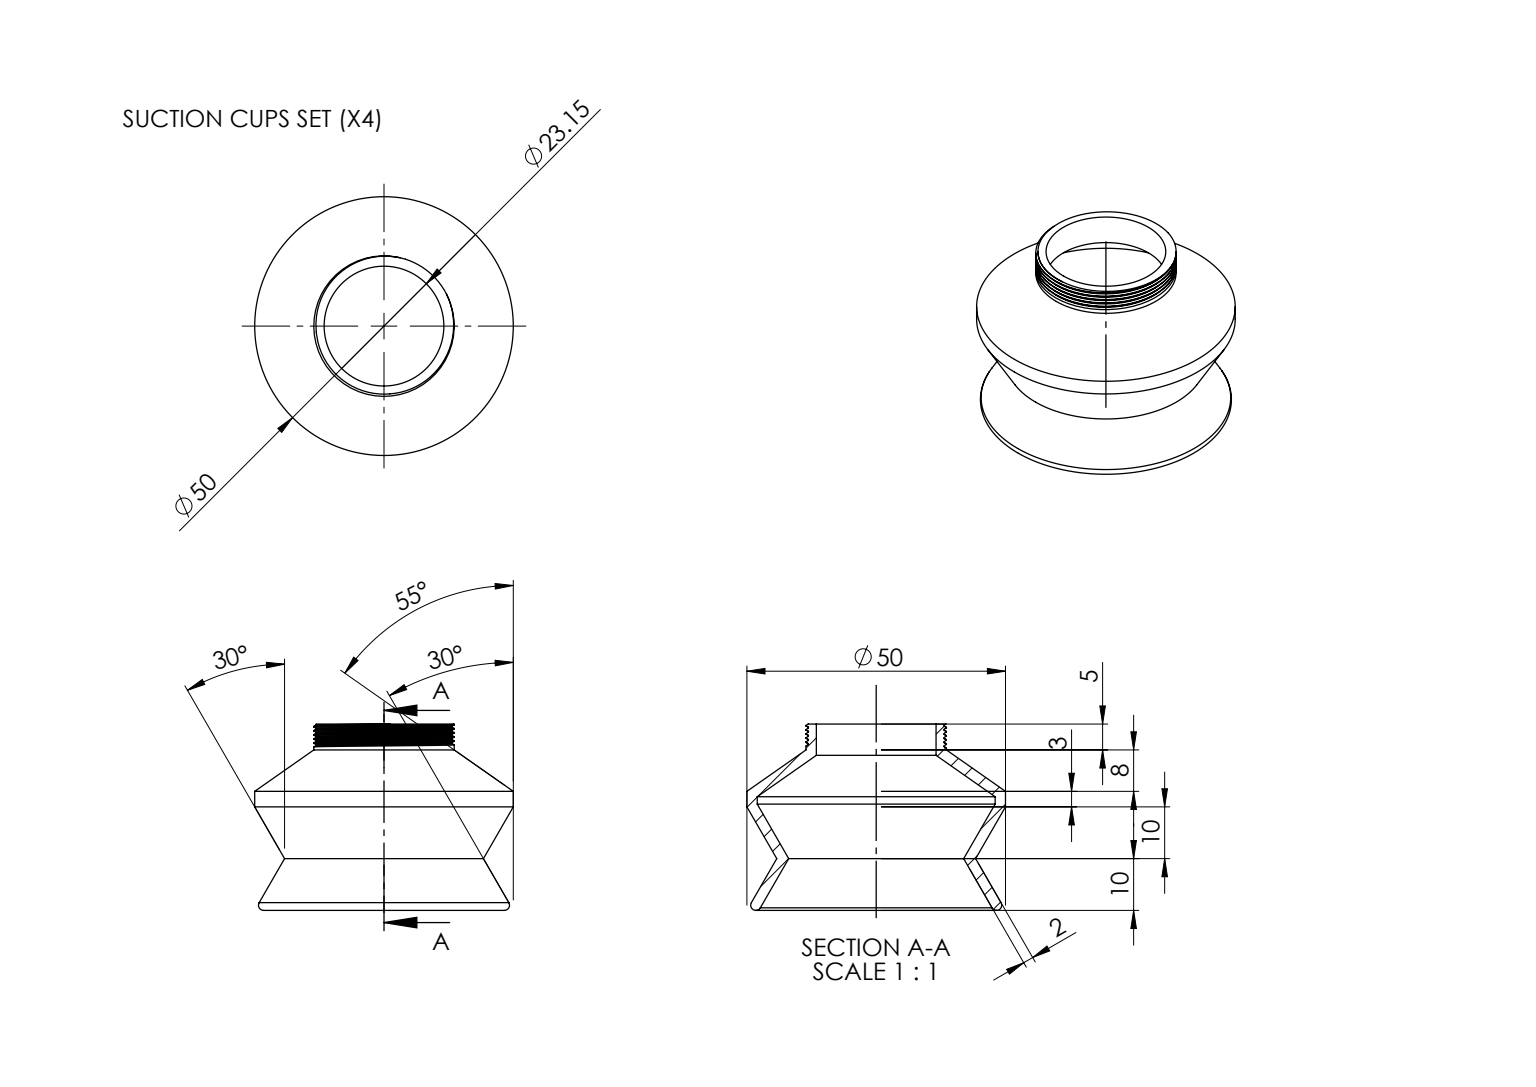
ISO-10303-21;
HEADER;
FILE_DESCRIPTION (('STEP AP214'),
    '1' );
FILE_NAME ('Suction Cups Set (x4).step',
    '2026-10-01T14:18:43',
    ( '' ),
    ( '' ),
    'SwSTEP 2.0',
    'SolidWorks 2026',
    '' );
FILE_SCHEMA (( 'AUTOMOTIVE_DESIGN' ));
ENDSEC;

DATA;
#7=ORIENTED_EDGE ( 'NONE', *, *, #7284, .F. ) ;
#8=CARTESIAN_POINT ( 'NONE',  ( 13.57481594606304753, 32.71523437500000142, -5.622872871577873966 ) ) ;
#12=CARTESIAN_POINT ( 'NONE',  ( 13.14518615778179544, 34.00507812608393721, -1.609821015232357215E-15 ) ) ;
#13=CARTESIAN_POINT ( 'NONE',  ( -5.444914386472299306, 39.31328125108394289, 13.14518615778179722 ) ) ;
#36=( BOUNDED_CURVE ( )  B_SPLINE_CURVE ( 2, ( #22936, #3397, #12350, #21068, #12069, #998, #12204, #16222, #18653 ),
 .UNSPECIFIED., .F., .F. ) 
 B_SPLINE_CURVE_WITH_KNOTS ( ( 3, 2, 2, 2, 3 ),
 ( 0.5208333333333332593, 0.5312499999999997780, 0.5416666666666664076, 0.5520833333333330373, 0.5624999999999996669 ),
 .UNSPECIFIED. ) 
 CURVE ( )  GEOMETRIC_REPRESENTATION_ITEM ( )  RATIONAL_B_SPLINE_CURVE ( ( 1.000000000000000888, 0.9238795325112859613, 1.000000000000000000, 0.9238795325112867385, 1.000000000000000000, 0.9238795325112867385, 1.000000000000000000, 0.9238795325112891810, 0.9999999999999975575 ) ) 
 REPRESENTATION_ITEM ( '' )  );
#41=CYLINDRICAL_SURFACE ( 'NONE', #26554, 13.57481594606304576 ) ;
#45=ORIENTED_EDGE ( 'NONE', *, *, #19075, .T. ) ;
#47=AXIS2_PLACEMENT_3D ( 'NONE', #20882, #18604, #27308 ) ;
#48=CARTESIAN_POINT ( 'NONE',  ( -13.14518615778179900, 40.50390625108394005, -5.444914386472297529 ) ) ;
#88=EDGE_CURVE ( 'NONE', #26327, #25494, #13051, .T. ) ;
#90=SURFACE_STYLE_USAGE ( .BOTH. , #4222 ) ;
#97=CARTESIAN_POINT ( 'NONE',  ( 13.14518615778179544, 38.56914062608393579, -1.609821015232357215E-15 ) ) ;
#113=DIRECTION ( 'NONE',  ( 0.000000000000000000, 0.000000000000000000, 1.000000000000000000 ) ) ;
#124=CARTESIAN_POINT ( 'NONE',  ( 13.57481594606304576, 37.42812499999999432, -1.662435489736055892E-15 ) ) ;
#126=CARTESIAN_POINT ( 'NONE',  ( 5.444914386472297529, 36.53515625108393294, -13.14518615778179900 ) ) ;
#148=ORIENTED_EDGE ( 'NONE', *, *, #16828, .T. ) ;
#149=CARTESIAN_POINT ( 'NONE',  ( -8.312177448680279460E-16, 32.96328125216787441, -13.57481594606304576 ) ) ;
#154=CARTESIAN_POINT ( 'NONE',  ( 13.14518615778179544, 38.76757812608393294, -1.609821015232357215E-15 ) ) ;
#233=CARTESIAN_POINT ( 'NONE',  ( 5.444914386472297529, 38.71796875108393721, -13.14518615778179900 ) ) ;
#244=ORIENTED_EDGE ( 'NONE', *, *, #571, .T. ) ;
#252=VECTOR ( 'NONE', #26544, 1000.000000000000114 ) ;
#253=CARTESIAN_POINT ( 'NONE',  ( 6.106658654948486920, 35.99999999999996447, 11.74215035806527396 ) ) ;
#266=CARTESIAN_POINT ( 'NONE',  ( -13.57481594606304576, 38.61874999999999147, 0.000000000000000000 ) ) ;
#268=CARTESIAN_POINT ( 'NONE',  ( 13.14518615778179900, 38.02343750108395426, -5.444914386472297529 ) ) ;
#281=ORIENTED_EDGE ( 'NONE', *, *, #3794, .F. ) ;
#285=TOROIDAL_SURFACE ( 'NONE', #12557, 23.26794919243112858, 1.000000000000000000 ) ;
#297=CARTESIAN_POINT ( 'NONE',  ( -9.295050272127046043, 39.06523437608392868, -9.295050272127046043 ) ) ;
#331=CARTESIAN_POINT ( 'NONE',  ( 13.14518615778179900, 38.51953125108393294, 5.444914386472293977 ) ) ;
#365=CARTESIAN_POINT ( 'NONE',  ( 2.493653234604083739E-15, 35.64218749999999147, 13.57481594606304576 ) ) ;
#380=CARTESIAN_POINT ( 'NONE',  ( -9.295050272127046043, 40.45429687608393721, -9.295050272127046043 ) ) ;
#391=ORIENTED_EDGE ( 'NONE', *, *, #1518, .F. ) ;
#399=ORIENTED_EDGE ( 'NONE', *, *, #6701, .T. ) ;
#400=CARTESIAN_POINT ( 'NONE',  ( 3.304118597822780057, 36.00000000000001421, 12.77244747738236441 ) ) ;
#409=CARTESIAN_POINT ( 'NONE',  ( -5.622872871578057818, 35.59257812499998863, 13.57481594606286457 ) ) ;
#411=CARTESIAN_POINT ( 'NONE',  ( -5.622872871577873077, 37.97382812499999716, 13.57481594606304753 ) ) ;
#413=CARTESIAN_POINT ( 'NONE',  ( -8.049105076161786076E-16, 36.58476562608393579, -13.14518615778179544 ) ) ;
#437=CARTESIAN_POINT ( 'NONE',  ( 5.444914386472297529, 35.74140625108393721, -13.14518615778179900 ) ) ;
#451=EDGE_CURVE ( 'NONE', #10079, #19989, #7039, .T. ) ;
#472=ORIENTED_EDGE ( 'NONE', *, *, #2653, .T. ) ;
#474=CARTESIAN_POINT ( 'NONE',  ( -13.14518615778179189, 39.01562500108393294, 5.444914386472304635 ) ) ;
#522=CARTESIAN_POINT ( 'NONE',  ( 13.14518615778179544, 35.39414062608393152, -1.609821015232357215E-15 ) ) ;
#554=CARTESIAN_POINT ( 'NONE',  ( 5.622872871577878406, 37.27929687499999289, 13.57481594606304576 ) ) ;
#555=CARTESIAN_POINT ( 'NONE',  ( -2.086998648631069653, 36.00000000000000000, -13.31420566034952202 ) ) ;
#556=CARTESIAN_POINT ( 'NONE',  ( -8.049105076161786076E-16, 33.40976562608393863, -13.14518615778179544 ) ) ;
#559=CARTESIAN_POINT ( 'NONE',  ( 9.598844408820459861, 35.04687500216787299, 9.598844408820456309 ) ) ;
#571=EDGE_CURVE ( 'NONE', #4666, #18529, #26293, .T. ) ;
#580=DIRECTION ( 'NONE',  ( 0.000000000000000000, 0.000000000000000000, -1.000000000000000000 ) ) ;
#584=CARTESIAN_POINT ( 'NONE',  ( -5.444914386472299306, 35.34453125108393579, 13.14518615778179722 ) ) ;
#615=CARTESIAN_POINT ( 'NONE',  ( 13.14518615778179900, 36.23750000108393010, -5.444914386472297529 ) ) ;
#645=ORIENTED_EDGE ( 'NONE', *, *, #3764, .T. ) ;
#658=CARTESIAN_POINT ( 'NONE',  ( -9.598844408820454532, 34.05468750216788010, 9.598844408820459861 ) ) ;
#660=ORIENTED_EDGE ( 'NONE', *, *, #2653, .F. ) ;
#664=CARTESIAN_POINT ( 'NONE',  ( -5.622872871577920151, 35.39414062716787868, -13.57481594606300135 ) ) ;
#667=CARTESIAN_POINT ( 'NONE',  ( -5.444914386472297529, 37.22968750108393721, -13.14518615778179900 ) ) ;
#690=CARTESIAN_POINT ( 'NONE',  ( -8.312177448680279460E-16, 37.72578125216787726, -13.57481594606304576 ) ) ;
#696=CARTESIAN_POINT ( 'NONE',  ( -9.598844408820458085, 35.34453124999998863, -9.598844408820458085 ) ) ;
#698=CARTESIAN_POINT ( 'NONE',  ( 5.622872871577878406, 34.10429687499999574, 13.57481594606304576 ) ) ;
#700=CARTESIAN_POINT ( 'NONE',  ( -13.14518615778179900, 33.55859375108393294, -5.444914386472297529 ) ) ;
#702=CARTESIAN_POINT ( 'NONE',  ( -9.295050272127044266, 35.09648437608392868, 9.295050272127047819 ) ) ;
#703=CARTESIAN_POINT ( 'NONE',  ( -5.622872871577873077, 34.89804687716787868, 13.57481594606304753 ) ) ;
#721=VECTOR ( 'NONE', #26504, 1000.000000000000000 ) ;
#727=CARTESIAN_POINT ( 'NONE',  ( 13.14518615778179900, 36.43593750108392726, -5.444914386472297529 ) ) ;
#733=EDGE_CURVE ( 'NONE', #12114, #10399, #2983, .T. ) ;
#743=AXIS2_PLACEMENT_3D ( 'NONE', #5650, #23447, #6063 ) ;
#750=DIRECTION ( 'NONE',  ( -1.000000000000000000, 0.000000000000000000, 0.000000000000000000 ) ) ;
#758=CARTESIAN_POINT ( 'NONE',  ( -13.14518615778179189, 35.04687500108393294, 5.444914386472304635 ) ) ;
#794=( BOUNDED_CURVE ( )  B_SPLINE_CURVE ( 2, ( #5981, #8244, #25772, #1851, #19221, #27923, #21502, #17214, #25918 ),
 .UNSPECIFIED., .F., .T. ) 
 B_SPLINE_CURVE_WITH_KNOTS ( ( 3, 2, 2, 2, 3 ),
 ( 0.5249747582430949189, 0.5312500000000001110, 0.5416666666666668517, 0.5520833333333337034, 0.5625000000000004441 ),
 .UNSPECIFIED. ) 
 CURVE ( )  GEOMETRIC_REPRESENTATION_ITEM ( )  RATIONAL_B_SPLINE_CURVE ( ( 0.9635368518655842429, 0.9541432637305302666, 1.000000000000000000, 0.9238795325112867385, 1.000000000000000000, 0.9238795325112867385, 1.000000000000000000, 0.9238795325112835188, 1.000000000000003331 ) ) 
 REPRESENTATION_ITEM ( '' )  );
#813=CARTESIAN_POINT ( 'NONE',  ( 2.414731522848535132E-15, 35.98945312608393010, 13.14518615778179544 ) ) ;
#837=CARTESIAN_POINT ( 'NONE',  ( -13.57481594606304576, 38.76757812716787299, 5.622872871577880183 ) ) ;
#845=CARTESIAN_POINT ( 'NONE',  ( -9.598844408820458085, 33.75703124999999005, -9.598844408820458085 ) ) ;
#847=CARTESIAN_POINT ( 'NONE',  ( 2.414731522848535132E-15, 35.39414062608393863, 13.14518615778179544 ) ) ;
#849=CARTESIAN_POINT ( 'NONE',  ( -13.14518615778179189, 34.25312500108393721, 5.444914386472304635 ) ) ;
#851=CARTESIAN_POINT ( 'NONE',  ( 13.57481594606304576, 35.14609375216787157, -1.662435489736055892E-15 ) ) ;
#876=CARTESIAN_POINT ( 'NONE',  ( -5.444914386472299306, 36.93203125108394147, 13.14518615778179722 ) ) ;
#906=CARTESIAN_POINT ( 'NONE',  ( 5.444914386472297529, 35.54296875108393294, -13.14518615778179900 ) ) ;
#908=CARTESIAN_POINT ( 'NONE',  ( 0.000000000000000000, 11.00000000000000355, 0.000000000000000000 ) ) ;
#909=CIRCLE ( 'NONE', #6776, 11.57481594606304576 ) ;
#963=ORIENTED_EDGE ( 'NONE', *, *, #21718, .F. ) ;
#977=CARTESIAN_POINT ( 'NONE',  ( 5.444914386472302859, 32.26875000108393721, 13.14518615778179189 ) ) ;
#980=CARTESIAN_POINT ( 'NONE',  ( -13.57481594606304576, 38.71796875216787726, 0.000000000000000000 ) ) ;
#984=EDGE_CURVE ( 'NONE', #27010, #13376, #11532, .T. ) ;
#988=CARTESIAN_POINT ( 'NONE',  ( 9.598844408820456309, 32.76484374999999716, -9.598844408820458085 ) ) ;
#990=CARTESIAN_POINT ( 'NONE',  ( 13.14518615778179544, 35.59257812608393579, -1.609821015232357215E-15 ) ) ;
#992=CARTESIAN_POINT ( 'NONE',  ( 9.295050272127046043, 35.49335937608393010, -9.295050272127046043 ) ) ;
#993=CARTESIAN_POINT ( 'NONE',  ( 13.57481594606304753, 36.78320312716786589, -5.622872871577873077 ) ) ;
#998=CARTESIAN_POINT ( 'NONE',  ( 13.57481594606304931, 35.09648437716787583, 5.622872871577868636 ) ) ;
#1019=CARTESIAN_POINT ( 'NONE',  ( 13.14518615778179900, 37.92421875108392726, 5.444914386472293977 ) ) ;
#1029=CARTESIAN_POINT ( 'NONE',  ( -5.622872871578010745, 32.91367187499999858, -13.57481594606290898 ) ) ;
#1048=CARTESIAN_POINT ( 'NONE',  ( -5.444914386472299306, 35.93984375108392726, 13.14518615778179722 ) ) ;
#1107=EDGE_LOOP ( 'NONE', ( #12800, #23533, #16863, #391 ) ) ;
#1116=CARTESIAN_POINT ( 'NONE',  ( 13.14518615778179722, 32.36796875108393579, 5.444914386472293977 ) ) ;
#1120=CARTESIAN_POINT ( 'NONE',  ( -9.598844408820454532, 39.61093750216787868, 9.598844408820459861 ) ) ;
#1121=CARTESIAN_POINT ( 'NONE',  ( 0.000000000000000000, 36.00000000000000000, 0.000000000000000000 ) ) ;
#1123=CARTESIAN_POINT ( 'NONE',  ( 2.493653234604083739E-15, 33.36015625216786873, 13.57481594606304576 ) ) ;
#1128=CARTESIAN_POINT ( 'NONE',  ( 13.57481594606304931, 34.99726562500000426, 5.622872871577869525 ) ) ;
#1130=CARTESIAN_POINT ( 'NONE',  ( -13.14518615778179544, 33.60820312608393579, 0.000000000000000000 ) ) ;
#1133=CARTESIAN_POINT ( 'NONE',  ( -8.049105076161786076E-16, 35.59257812608393579, -13.14518615778179544 ) ) ;
#1134=CARTESIAN_POINT ( 'NONE',  ( 9.598844408820456309, 35.24531250216787726, -9.598844408820458085 ) ) ;
#1138=ADVANCED_FACE ( 'NONE', ( #11527 ), #24418, .T. ) ;
#1139=( BOUNDED_CURVE ( )  B_SPLINE_CURVE ( 2, ( #3619, #1763, #16297, #14700, #12004, #8164, #16721, #14147, #25418 ),
 .UNSPECIFIED., .F., .F. ) 
 B_SPLINE_CURVE_WITH_KNOTS ( ( 3, 2, 2, 2, 3 ),
 ( 0.8541666666666670737, 0.8645833333333337034, 0.8750000000000003331, 0.8854166666666669627, 0.8958333333333335924 ),
 .UNSPECIFIED. ) 
 CURVE ( )  GEOMETRIC_REPRESENTATION_ITEM ( )  RATIONAL_B_SPLINE_CURVE ( ( 0.9999999999999967804, 0.9238795325112899581, 1.000000000000000000, 0.9238795325112867385, 1.000000000000000000, 0.9238795325112867385, 1.000000000000000000, 0.9238795325112850731, 1.000000000000001554 ) ) 
 REPRESENTATION_ITEM ( '' )  );
#1148=DIRECTION ( 'NONE',  ( -0.000000000000000000, -1.000000000000000000, -0.000000000000000000 ) ) ;
#1160=CARTESIAN_POINT ( 'NONE',  ( -5.444914386472299306, 32.16953125108393152, 13.14518615778179722 ) ) ;
#1183=AXIS2_PLACEMENT_3D ( 'NONE', #15127, #17283, #25985 ) ;
#1191=CARTESIAN_POINT ( 'NONE',  ( -9.295050272127046043, 35.69179687608393436, -9.295050272127046043 ) ) ;
#1199=CARTESIAN_POINT ( 'NONE',  ( 0.000000000000000000, -1.000000000000001998, 23.26794919243113213 ) ) ;
#1215=CARTESIAN_POINT ( 'NONE',  ( -5.622872871577828668, 33.21132812499999432, 13.57481594606309194 ) ) ;
#1217=ORIENTED_EDGE ( 'NONE', *, *, #20623, .T. ) ;
#1238=CARTESIAN_POINT ( 'NONE',  ( -13.14518615778179544, 39.95820312608393010, 0.000000000000000000 ) ) ;
#1264=CARTESIAN_POINT ( 'NONE',  ( -13.57481594606304753, 33.01289062500000426, -5.622872871577873077 ) ) ;
#1266=CARTESIAN_POINT ( 'NONE',  ( 13.14518615778179900, 32.36796875108393579, 5.444914386472293977 ) ) ;
#1269=CARTESIAN_POINT ( 'NONE',  ( 13.57481594606304753, 33.60820312716787583, -5.622872871577873077 ) ) ;
#1290=CARTESIAN_POINT ( 'NONE',  ( 5.444914386472297529, 32.56640625108394005, -13.14518615778179900 ) ) ;
#1297=DIRECTION ( 'NONE',  ( 0.000000000000000000, 1.000000000000000000, 0.000000000000000000 ) ) ;
#1319=CARTESIAN_POINT ( 'NONE',  ( 0.000000000000000000, 36.00000000000000000, -13.57481594606304576 ) ) ;
#1321=EDGE_CURVE ( 'NONE', #8614, #8271, #20654, .T. ) ;
#1324=CARTESIAN_POINT ( 'NONE',  ( 5.444914386472302859, 32.07031250108393294, 13.14518615778179189 ) ) ;
#1340=CARTESIAN_POINT ( 'NONE',  ( 5.444914386472302859, 35.24531250108393010, 13.14518615778179189 ) ) ;
#1348=CARTESIAN_POINT ( 'NONE',  ( 0.000000000000000000, 23.00000000000000000, 0.000000000000000000 ) ) ;
#1364=ADVANCED_FACE ( 'NONE', ( #11468 ), #9382, .T. ) ;
#1374=CARTESIAN_POINT ( 'NONE',  ( -8.312177448680279460E-16, 34.55078125216787299, -13.57481594606304576 ) ) ;
#1376=CARTESIAN_POINT ( 'NONE',  ( 13.14518615778179900, 39.51171875108392584, 5.444914386472293977 ) ) ;
#1378=DIRECTION ( 'NONE',  ( 0.000000000000000000, 0.000000000000000000, -1.000000000000000000 ) ) ;
#1396=CARTESIAN_POINT ( 'NONE',  ( -13.57481594606304753, 33.80664062499999289, -5.622872871577872189 ) ) ;
#1407=CARTESIAN_POINT ( 'NONE',  ( -11.14554687309540348, 36.00000000000000711, -7.260818043107225783 ) ) ;
#1408=CARTESIAN_POINT ( 'NONE',  ( -8.312177448680279460E-16, 39.21406249999999716, -13.57481594606304576 ) ) ;
#1409=CARTESIAN_POINT ( 'NONE',  ( -9.295050272127046043, 32.51679687608393721, -9.295050272127046043 ) ) ;
#1410=CARTESIAN_POINT ( 'NONE',  ( 13.57481594606304576, 31.97109375216787441, -1.662435489736055892E-15 ) ) ;
#1431=CARTESIAN_POINT ( 'NONE',  ( -13.14518615778179900, 33.55859375108393294, -5.444914386472297529 ) ) ;
#1436=AXIS2_PLACEMENT_3D ( 'NONE', #21286, #10435, #12707 ) ;
#1464=CARTESIAN_POINT ( 'NONE',  ( -13.14518615778179900, 34.94765625108392726, -5.444914386472297529 ) ) ;
#1478=CARTESIAN_POINT ( 'NONE',  ( 9.295050272127046043, 33.90585937608393152, -9.295050272127046043 ) ) ;
#1499=AXIS2_PLACEMENT_3D ( 'NONE', #4264, #19936, #23788 ) ;
#1506=VERTEX_POINT ( 'NONE', #23202 ) ;
#1509=CARTESIAN_POINT ( 'NONE',  ( 9.598844408820456309, 33.65781250216787157, -9.598844408820458085 ) ) ;
#1518=EDGE_CURVE ( 'NONE', #12537, #26666, #15283, .T. ) ;
#1549=CARTESIAN_POINT ( 'NONE',  ( 9.598844408820456309, 39.11484374999999858, -9.598844408820458085 ) ) ;
#1550=CARTESIAN_POINT ( 'NONE',  ( 13.14518615778179544, 33.80664062608393294, -1.609821015232357215E-15 ) ) ;
#1551=CARTESIAN_POINT ( 'NONE',  ( -5.622872871577873077, 32.21914062716787441, -13.57481594606304753 ) ) ;
#1570=ORIENTED_EDGE ( 'NONE', *, *, #18211, .T. ) ;
#1573=CARTESIAN_POINT ( 'NONE',  ( 2.414731522848535132E-15, 33.01289062608393721, 13.14518615778179544 ) ) ;
#1591=CARTESIAN_POINT ( 'NONE',  ( -10.78684676818415689, 36.00000000000000000, 7.561388982944556858 ) ) ;
#1603=CARTESIAN_POINT ( 'NONE',  ( -13.14518615778179189, 34.25312500108393010, 5.444914386472304635 ) ) ;
#1617=CARTESIAN_POINT ( 'NONE',  ( 9.295050272127046043, 32.31835937608393294, -9.295050272127046043 ) ) ;
#1620=ORIENTED_EDGE ( 'NONE', *, *, #6276, .F. ) ;
#1670=CARTESIAN_POINT ( 'NONE',  ( -8.312177448680279460E-16, 33.65781249999999147, -13.57481594606304576 ) ) ;
#1679=CARTESIAN_POINT ( 'NONE',  ( 3.878385297391210518, 32.03609435653363136, -13.57481594606304576 ) ) ;
#1681=CARTESIAN_POINT ( 'NONE',  ( 13.14518615778179900, 32.46718750108393436, -5.444914386472297529 ) ) ;
#1682=CARTESIAN_POINT ( 'NONE',  ( 13.14518615778179722, 32.96328125108393436, 5.444914386472293977 ) ) ;
#1684=CARTESIAN_POINT ( 'NONE',  ( -13.57481594606304576, 32.36796875216787583, 0.000000000000000000 ) ) ;
#1739=CARTESIAN_POINT ( 'NONE',  ( -13.14518615778179900, 33.36015625108393579, -5.444914386472297529 ) ) ;
#1756=CARTESIAN_POINT ( 'NONE',  ( -13.14518615778179900, 34.15390625108393863, -5.444914386472297529 ) ) ;
#1763=CARTESIAN_POINT ( 'NONE',  ( 5.622872871578054266, 32.11992187716787583, -13.57481594606286635 ) ) ;
#1811=CONICAL_SURFACE ( 'NONE', #27315, 17.49444650053485972, 0.5235987755983000369 ) ;
#1818=CARTESIAN_POINT ( 'NONE',  ( -13.57481594606304753, 40.15664062500000142, -5.622872871577873077 ) ) ;
#1819=CARTESIAN_POINT ( 'NONE',  ( -13.14518615778179189, 31.87187500108393223, 5.444914386472304635 ) ) ;
#1820=AXIS2_PLACEMENT_3D ( 'NONE', #15006, #28143, #23728 ) ;
#1821=CARTESIAN_POINT ( 'NONE',  ( -5.622872871577873077, 32.51679687716787726, 13.57481594606304753 ) ) ;
#1827=( BOUNDED_CURVE ( )  B_SPLINE_CURVE ( 2, ( #15862, #22440, #22726, #22583, #26575, #3052, #24425, #24284, #5053 ),
 .UNSPECIFIED., .F., .T. ) 
 B_SPLINE_CURVE_WITH_KNOTS ( ( 3, 2, 2, 2, 3 ),
 ( 0.6874999999999997780, 0.6979166666666665186, 0.7083333333333333703, 0.7187500000000001110, 0.7291666666666668517 ),
 .UNSPECIFIED. ) 
 CURVE ( )  GEOMETRIC_REPRESENTATION_ITEM ( )  RATIONAL_B_SPLINE_CURVE ( ( 1.000000000000001554, 0.9238795325112850731, 1.000000000000000000, 0.9238795325112867385, 1.000000000000000000, 0.9238795325112867385, 1.000000000000000000, 0.9238795325112850731, 1.000000000000001554 ) ) 
 REPRESENTATION_ITEM ( '' )  );
#1836=EDGE_CURVE ( 'NONE', #22508, #6997, #16140, .T. ) ;
#1841=CONICAL_SURFACE ( 'NONE', #10015, 19.22649730810373470, 0.5235987755983000369 ) ;
#1851=CARTESIAN_POINT ( 'NONE',  ( 13.57481594606304753, 35.89023437499999858, -5.622872871577873966 ) ) ;
#1864=CARTESIAN_POINT ( 'NONE',  ( -12.37587840034922770, 35.99999999999998579, 4.513979326318623642 ) ) ;
#1867=ORIENTED_EDGE ( 'NONE', *, *, #16501, .T. ) ;
#1869=DIRECTION ( 'NONE',  ( -0.000000000000000000, -1.000000000000000000, -0.000000000000000000 ) ) ;
#1870=ORIENTED_EDGE ( 'NONE', *, *, #22385, .F. ) ;
#1881=CARTESIAN_POINT ( 'NONE',  ( -9.295050272127046043, 34.10429687608393579, -9.295050272127046043 ) ) ;
#1897=CARTESIAN_POINT ( 'NONE',  ( -8.049105076161786076E-16, 33.21132812608393436, -13.14518615778179544 ) ) ;
#1955=CARTESIAN_POINT ( 'NONE',  ( 5.444914386472297529, 32.36796875108393579, -13.14518615778179722 ) ) ;
#1957=CARTESIAN_POINT ( 'NONE',  ( 9.295050272127047819, 39.26367187608393294, 9.295050272127046043 ) ) ;
#1978=EDGE_LOOP ( 'NONE', ( #4745, #16470, #24296, #6881 ) ) ;
#1988=CARTESIAN_POINT ( 'NONE',  ( -9.295050272127046043, 38.27148437608393294, -9.295050272127046043 ) ) ;
#1997=CARTESIAN_POINT ( 'NONE',  ( -4.780039198850967175, 35.99999999999999289, 12.25280873422855699 ) ) ;
#2011=CARTESIAN_POINT ( 'NONE',  ( 13.14518615778179900, 38.71796875108393721, 5.444914386472293977 ) ) ;
#2025=CONICAL_SURFACE ( 'NONE', #17016, 23.26794919243113213, 0.5235987755983000369 ) ;
#2028=CYLINDRICAL_SURFACE ( 'NONE', #12076, 13.57481594606304576 ) ;
#2030=CARTESIAN_POINT ( 'NONE',  ( 9.295050272127047819, 32.11992187608393579, 9.295050272127046043 ) ) ;
#2039=CARTESIAN_POINT ( 'NONE',  ( 0.000000000000000000, -1.000000000000001998, 0.000000000000000000 ) ) ;
#2048=CARTESIAN_POINT ( 'NONE',  ( 5.444914386472302859, 39.21406250108392300, 13.14518615778179189 ) ) ;
#2082=CARTESIAN_POINT ( 'NONE',  ( -9.295050272127046043, 33.50898437608393010, -9.295050272127046043 ) ) ;
#2094=CARTESIAN_POINT ( 'NONE',  ( 5.444914386472302859, 39.21406250108392300, 13.14518615778179189 ) ) ;
#2122=DIRECTION ( 'NONE',  ( 0.000000000000000000, 1.000000000000000000, 0.000000000000000000 ) ) ;
#2124=CARTESIAN_POINT ( 'NONE',  ( -13.57481594606304576, 36.28710937499999289, 5.622872871577880183 ) ) ;
#2125=CARTESIAN_POINT ( 'NONE',  ( 0.000000000000000000, 23.00000000000000000, -25.00000000000001066 ) ) ;
#2127=CARTESIAN_POINT ( 'NONE',  ( -8.049105076161786076E-16, 38.96601562608393721, -13.14518615778179544 ) ) ;
#2141=VECTOR ( 'NONE', #25293, 1000.000000000000000 ) ;
#2153=CARTESIAN_POINT ( 'NONE',  ( -9.295050272127046043, 34.30273437608393294, -9.295050272127046043 ) ) ;
#2154=CARTESIAN_POINT ( 'NONE',  ( -13.14518615778179189, 38.42031250108393436, 5.444914386472304635 ) ) ;
#2155=UNCERTAINTY_MEASURE_WITH_UNIT (LENGTH_MEASURE( 1.000000000000000082E-05 ), #19187, 'distance_accuracy_value', 'NONE');
#2184=CARTESIAN_POINT ( 'NONE',  ( 0.000000000000000000, 29.95886589889650509, 0.000000000000000000 ) ) ;
#2190=CARTESIAN_POINT ( 'NONE',  ( 13.14518615778179900, 40.10703125108393152, 5.444914386472293977 ) ) ;
#2194=DIRECTION ( 'NONE',  ( -0.000000000000000000, -1.000000000000000000, -0.000000000000000000 ) ) ;
#2205=EDGE_CURVE ( 'NONE', #8864, #26666, #22169, .T. ) ;
#2237=ORIENTED_EDGE ( 'NONE', *, *, #16828, .F. ) ;
#2241=CARTESIAN_POINT ( 'NONE',  ( -13.14518615778179189, 39.01562500108393294, 5.444914386472304635 ) ) ;
#2272=CARTESIAN_POINT ( 'NONE',  ( -13.57481594606304576, 37.82499999999999574, 0.000000000000000000 ) ) ;
#2274=CARTESIAN_POINT ( 'NONE',  ( -9.295050272127044266, 37.67617187608393436, 9.295050272127047819 ) ) ;
#2299=CARTESIAN_POINT ( 'NONE',  ( 9.295050272127046043, 35.69179687608394147, -9.295050272127046043 ) ) ;
#2300=CARTESIAN_POINT ( 'NONE',  ( 13.14518615778179900, 39.51171875108392584, 5.444914386472293977 ) ) ;
#2332=CARTESIAN_POINT ( 'NONE',  ( 2.414731522848535132E-15, 39.95820312608393010, 13.14518615778179544 ) ) ;
#2365=FACE_OUTER_BOUND ( 'NONE', #26834, .T. ) ;
#2370=CARTESIAN_POINT ( 'NONE',  ( 1.662435489736055892E-15, 36.00000000000000000, 13.57481594606304576 ) ) ;
#2376=PRESENTATION_STYLE_ASSIGNMENT (( #90 ) ) ;
#2383=CARTESIAN_POINT ( 'NONE',  ( -5.444914386472299306, 39.90859375108393436, 13.14518615778179722 ) ) ;
#2413=CARTESIAN_POINT ( 'NONE',  ( -13.57481594606304576, 36.23749999999999005, 0.000000000000000000 ) ) ;
#2415=CARTESIAN_POINT ( 'NONE',  ( -9.295050272127044266, 36.88242187608393152, 9.295050272127047819 ) ) ;
#2439=CARTESIAN_POINT ( 'NONE',  ( -5.444914386472297529, 33.45937500108394147, -13.14518615778179722 ) ) ;
#2440=CARTESIAN_POINT ( 'NONE',  ( 2.414731522848535132E-15, 39.36289062608393152, 13.14518615778179544 ) ) ;
#2459=FACE_OUTER_BOUND ( 'NONE', #14459, .T. ) ;
#2467=EDGE_LOOP ( 'NONE', ( #15603, #6608, #7902, #4181 ) ) ;
#2472=CARTESIAN_POINT ( 'NONE',  ( 0.000000000000000000, 36.00000000000000000, -13.57481594606304576 ) ) ;
#2516=CARTESIAN_POINT ( 'NONE',  ( 2.414731522848535132E-15, 37.57695312608392868, 13.14518615778179544 ) ) ;
#2529=CARTESIAN_POINT ( 'NONE',  ( 13.57481594606304753, 33.50898437499999716, -5.622872871577873966 ) ) ;
#2536=EDGE_CURVE ( 'NONE', #13023, #4040, #19160, .T. ) ;
#2537=ORIENTED_EDGE ( 'NONE', *, *, #17851, .F. ) ;
#2540=CARTESIAN_POINT ( 'NONE',  ( 13.49550141231711287, 36.00000000000000711, -0.9550757908102345262 ) ) ;
#2551=CARTESIAN_POINT ( 'NONE',  ( -5.622872871577828668, 32.51679687716787015, 13.57481594606309194 ) ) ;
#2552=CARTESIAN_POINT ( 'NONE',  ( -9.598844408820458085, 36.13828124999999147, -9.598844408820458085 ) ) ;
#2554=CARTESIAN_POINT ( 'NONE',  ( 13.14518615778179900, 37.22968750108393721, -5.444914386472297529 ) ) ;
#2568=CARTESIAN_POINT ( 'NONE',  ( 13.57481594606304931, 34.99726562500000426, 5.622872871577868636 ) ) ;
#2582=CARTESIAN_POINT ( 'NONE',  ( 2.414731522848535132E-15, 40.15664062608393436, 13.14518615778179544 ) ) ;
#2612=CARTESIAN_POINT ( 'NONE',  ( -8.049105076161786076E-16, 40.35507812608393152, -13.14518615778179544 ) ) ;
#2649=LINE ( 'NONE', #4930, #20620 ) ;
#2653=EDGE_CURVE ( 'NONE', #8637, #10079, #11194, .T. ) ;
#2661=CARTESIAN_POINT ( 'NONE',  ( 9.295050272127047819, 36.88242187608393152, 9.295050272127046043 ) ) ;
#2683=CARTESIAN_POINT ( 'NONE',  ( 0.000000000000000000, 20.53589838486225361, 0.000000000000000000 ) ) ;
#2692=CARTESIAN_POINT ( 'NONE',  ( 9.598844408820456309, 37.52734375000000000, -9.598844408820458085 ) ) ;
#2693=CARTESIAN_POINT ( 'NONE',  ( 3.089260913797906571, 36.00000000000000000, -13.21136010216355672 ) ) ;
#2694=CARTESIAN_POINT ( 'NONE',  ( 5.444914386472302859, 33.06250000108393294, 13.14518615778179189 ) ) ;
#2698=CARTESIAN_POINT ( 'NONE',  ( -9.598844408820454532, 36.43593750216787441, 9.598844408820459861 ) ) ;
#2714=VECTOR ( 'NONE', #22615, 1000.000000000000000 ) ;
#2723=CARTESIAN_POINT ( 'NONE',  ( -9.295050272127044266, 36.88242187608393152, 9.295050272127047819 ) ) ;
#2751=AXIS2_PLACEMENT_3D ( 'NONE', #27587, #14727, #10734 ) ;
#2754=CARTESIAN_POINT ( 'NONE',  ( 13.14518615778179900, 37.72578125108393721, 5.444914386472293977 ) ) ;
#2783=( BOUNDED_CURVE ( )  B_SPLINE_CURVE ( 2, ( #14333, #8593, #5668, #19428, #23848, #1396, #12048, #18634, #1670 ),
 .UNSPECIFIED., .F., .F. ) 
 B_SPLINE_CURVE_WITH_KNOTS ( ( 3, 2, 2, 2, 3 ),
 ( 0.7291666666666668517, 0.7395833333333334814, 0.7500000000000001110, 0.7604166666666667407, 0.7708333333333333703 ),
 .UNSPECIFIED. ) 
 CURVE ( )  GEOMETRIC_REPRESENTATION_ITEM ( )  RATIONAL_B_SPLINE_CURVE ( ( 0.9999999999999983347, 0.9238795325112884038, 1.000000000000000000, 0.9238795325112867385, 1.000000000000000000, 0.9238795325112867385, 1.000000000000000000, 0.9238795325112867385, 1.000000000000000000 ) ) 
 REPRESENTATION_ITEM ( '' )  );
#2796=CYLINDRICAL_SURFACE ( 'NONE', #14411, 25.00000000000001066 ) ;
#2797=CARTESIAN_POINT ( 'NONE',  ( 5.444914386472302859, 34.45156250108393436, 13.14518615778179189 ) ) ;
#2804=DIRECTION ( 'NONE',  ( -0.8490667072653959035, 1.618318251311064231E-06, -0.5282856486891157610 ) ) ;
#2808=CARTESIAN_POINT ( 'NONE',  ( 5.622872871577924592, 33.31054687499999289, 13.57481594606299957 ) ) ;
#2818=DIRECTION ( 'NONE',  ( 0.000000000000000000, 0.000000000000000000, 1.000000000000000000 ) ) ;
#2819=CARTESIAN_POINT ( 'NONE',  ( -8.312177448680279460E-16, 38.51953125216787299, -13.57481594606304576 ) ) ;
#2825=ORIENTED_EDGE ( 'NONE', *, *, #3764, .F. ) ;
#2826=CARTESIAN_POINT ( 'NONE',  ( -5.622872871577782483, 35.29492187499999289, -13.57481594606313990 ) ) ;
#2828=CARTESIAN_POINT ( 'NONE',  ( -13.57481594606304576, 34.69960937499999432, 5.622872871577880183 ) ) ;
#2830=CARTESIAN_POINT ( 'NONE',  ( 13.14518615778179900, 34.05468750108394005, -5.444914386472297529 ) ) ;
#2833=CARTESIAN_POINT ( 'NONE',  ( -13.57481594606304753, 35.49335937716787015, -5.622872871577873077 ) ) ;
#2851=CARTESIAN_POINT ( 'NONE',  ( 9.598844408820456309, 32.86406250216787583, -9.598844408820458085 ) ) ;
#2856=CARTESIAN_POINT ( 'NONE',  ( 13.14518615778179900, 37.22968750108393721, -5.444914386472297529 ) ) ;
#2859=CARTESIAN_POINT ( 'NONE',  ( -8.312177448680279460E-16, 32.07031249999999289, -13.57481594606304576 ) ) ;
#2885=CARTESIAN_POINT ( 'NONE',  ( 9.295050272127047819, 36.88242187608393152, 9.295050272127046043 ) ) ;
#2898=CARTESIAN_POINT ( 'NONE',  ( 0.000000000000000000, 1.000000000000000000, 23.26794919243112858 ) ) ;
#2901=( BOUNDED_CURVE ( )  B_SPLINE_CURVE ( 2, ( #8242, #12224, #14780, #6114, #18535, #27239, #5573 ),
 .UNSPECIFIED., .F., .F. ) 
 B_SPLINE_CURVE_WITH_KNOTS ( ( 3, 2, 2, 3 ),
 ( 0.4520580917964582834, 0.4583333333333333148, 0.4687500000000000555, 0.4791666666666667962 ),
 .UNSPECIFIED. ) 
 CURVE ( )  GEOMETRIC_REPRESENTATION_ITEM ( )  RATIONAL_B_SPLINE_CURVE ( ( 0.9635368512068458458, 0.9541432653384140927, 1.000000000000000000, 0.9238795325112867385, 1.000000000000000000, 0.9238795325112859613, 1.000000000000000888 ) ) 
 REPRESENTATION_ITEM ( '' )  );
#2932=CARTESIAN_POINT ( 'NONE',  ( -8.049105076161786076E-16, 37.18007812608393436, -13.14518615778179544 ) ) ;
#2943=CARTESIAN_POINT ( 'NONE',  ( 5.622872871577870413, 33.60820312499999574, -13.57481594606304753 ) ) ;
#2955=CARTESIAN_POINT ( 'NONE',  ( -5.622872871577873077, 40.15664062716787441, -13.57481594606304753 ) ) ;
#2962=CARTESIAN_POINT ( 'NONE',  ( 13.57481594606304753, 32.71523437500000142, -5.622872871577873077 ) ) ;
#2963=CARTESIAN_POINT ( 'NONE',  ( 7.171390501253594785, 31.30502191632583830, -11.52591802191987114 ) ) ;
#2964=CARTESIAN_POINT ( 'NONE',  ( 9.295050272127046043, 34.89804687608393863, -9.295050272127046043 ) ) ;
#2966=CARTESIAN_POINT ( 'NONE',  ( -9.295050272127044266, 34.30273437608393294, 9.295050272127047819 ) ) ;
#2967=CARTESIAN_POINT ( 'NONE',  ( 9.598844408820459861, 37.42812500216787441, 9.598844408820456309 ) ) ;
#2983=( BOUNDED_CURVE ( )  B_SPLINE_CURVE ( 2, ( #3871, #4436, #12949 ),
 .UNSPECIFIED., .F., .F. ) 
 B_SPLINE_CURVE_WITH_KNOTS ( ( 3, 3 ),
 ( 0.9375000000000000000, 0.9448586960708869054 ),
 .UNSPECIFIED. ) 
 CURVE ( )  GEOMETRIC_REPRESENTATION_ITEM ( )  RATIONAL_B_SPLINE_CURVE ( ( 1.000000000000000000, 0.9462258510377660192, 0.9684275648627984623 ) ) 
 REPRESENTATION_ITEM ( '' )  );
#2989=( GEOMETRIC_REPRESENTATION_CONTEXT ( 3 ) GLOBAL_UNCERTAINTY_ASSIGNED_CONTEXT ( ( #26087 ) ) GLOBAL_UNIT_ASSIGNED_CONTEXT ( ( #4325, #16347, #22916 ) ) REPRESENTATION_CONTEXT ( 'NONE', 'WORKASPACE' ) );
#2995=CARTESIAN_POINT ( 'NONE',  ( 5.444914386472302859, 37.03125000108393294, 13.14518615778179189 ) ) ;
#2999=CARTESIAN_POINT ( 'NONE',  ( -13.57481594606304576, 32.26874999999999716, 0.000000000000000000 ) ) ;
#3004=CYLINDRICAL_SURFACE ( 'NONE', #25512, 13.57481594606304576 ) ;
#3028=CARTESIAN_POINT ( 'NONE',  ( 5.444914386472302859, 36.03906250108394005, 13.14518615778179189 ) ) ;
#3052=CARTESIAN_POINT ( 'NONE',  ( 13.57481594606304931, 34.20351562499999432, 5.622872871577868636 ) ) ;
#3071=( BOUNDED_CURVE ( )  B_SPLINE_CURVE ( 2, ( #13512, #24360, #11230, #8436, #13656, #2568, #22371, #15660, #20094 ),
 .UNSPECIFIED., .F., .F. ) 
 B_SPLINE_CURVE_WITH_KNOTS ( ( 3, 2, 2, 2, 3 ),
 ( 0.6041666666666668517, 0.6145833333333334814, 0.6250000000000001110, 0.6354166666666667407, 0.6458333333333333703 ),
 .UNSPECIFIED. ) 
 CURVE ( )  GEOMETRIC_REPRESENTATION_ITEM ( )  RATIONAL_B_SPLINE_CURVE ( ( 0.9999999999999983347, 0.9238795325112884038, 1.000000000000000000, 0.9238795325112867385, 1.000000000000000000, 0.9238795325112867385, 1.000000000000000000, 0.9238795325112867385, 1.000000000000000000 ) ) 
 REPRESENTATION_ITEM ( '' )  );
#3080=DIRECTION ( 'NONE',  ( -6.123233995736778362E-17, -0.8660254037844380415, -0.5000000000000009992 ) ) ;
#3086=EDGE_CURVE ( 'NONE', #19447, #4040, #3515, .T. ) ;
#3103=CARTESIAN_POINT ( 'NONE',  ( -8.049105076161786076E-16, 33.40976562608393863, -13.14518615778179544 ) ) ;
#3114=CARTESIAN_POINT ( 'NONE',  ( 13.57481594606304576, 35.04687499999999289, -1.662435489736055892E-15 ) ) ;
#3116=CARTESIAN_POINT ( 'NONE',  ( -13.14518615778179900, 32.76484375108393010, -5.444914386472297529 ) ) ;
#3120=CARTESIAN_POINT ( 'NONE',  ( -13.57481594606304753, 36.28710937716787299, -5.622872871577873077 ) ) ;
#3127=ORIENTED_EDGE ( 'NONE', *, *, #27642, .F. ) ;
#3146=CARTESIAN_POINT ( 'NONE',  ( -5.444914386472299306, 36.13828125108393863, 13.14518615778179722 ) ) ;
#3147=APPLICATION_CONTEXT ( 'automotive_design' ) ;
#3173=CARTESIAN_POINT ( 'NONE',  ( 2.414731522848535132E-15, 37.57695312608392868, 13.14518615778179544 ) ) ;
#3174=VECTOR ( 'NONE', #19468, 1000.000000000000000 ) ;
#3195=AXIS2_PLACEMENT_3D ( 'NONE', #5511, #7486, #9902 ) ;
#3219=CARTESIAN_POINT ( 'NONE',  ( 12.07727640983550188, 36.00000000000000000, -6.197985357349471869 ) ) ;
#3241=ADVANCED_FACE ( 'NONE', ( #15115 ), #2025, .F. ) ;
#3243=CARTESIAN_POINT ( 'NONE',  ( -9.295050272127044266, 33.70742187608393436, 9.295050272127047819 ) ) ;
#3247=CARTESIAN_POINT ( 'NONE',  ( -8.312177448680279460E-16, 39.31328125216787583, -13.57481594606304576 ) ) ;
#3256=CARTESIAN_POINT ( 'NONE',  ( -13.57481594606304576, 33.11210937499999574, 5.622872871577880183 ) ) ;
#3257=CARTESIAN_POINT ( 'NONE',  ( -7.394032042335738630, 36.00000000000004263, -11.20317769887113180 ) ) ;
#3258=CARTESIAN_POINT ( 'NONE',  ( -13.14518615778179189, 33.65781250108393152, 5.444914386472304635 ) ) ;
#3261=CARTESIAN_POINT ( 'NONE',  ( -13.57481594606304576, 35.54296875216788010, 0.000000000000000000 ) ) ;
#3266=CARTESIAN_POINT ( 'NONE',  ( 0.000000000000000000, 10.00000000000000000, 0.000000000000000000 ) ) ;
#3282=ORIENTED_EDGE ( 'NONE', *, *, #451, .F. ) ;
#3283=CARTESIAN_POINT ( 'NONE',  ( 2.414731522848535132E-15, 32.21914062608393436, 13.14518615778179544 ) ) ;
#3314=CARTESIAN_POINT ( 'NONE',  ( -8.049105076161786076E-16, 36.38632812608393152, -13.14518615778179544 ) ) ;
#3325=CARTESIAN_POINT ( 'NONE',  ( -8.312177448680279460E-16, 33.65781249999999147, -13.57481594606304576 ) ) ;
#3329=VERTEX_POINT ( 'NONE', #11266 ) ;
#3359=CARTESIAN_POINT ( 'NONE',  ( 13.14518615778179900, 40.30546875108393579, 5.444914386472293977 ) ) ;
#3374=CARTESIAN_POINT ( 'NONE',  ( 5.444914386472297529, 33.36015625108393579, -13.14518615778179722 ) ) ;
#3386=CARTESIAN_POINT ( 'NONE',  ( 9.598844408820459861, 33.36015624999999574, 9.598844408820456309 ) ) ;
#3389=CARTESIAN_POINT ( 'NONE',  ( 9.295050272127046043, 32.51679687608393721, -9.295050272127046043 ) ) ;
#3391=CARTESIAN_POINT ( 'NONE',  ( 5.444914386472297529, 34.74921875108393721, -13.14518615778179722 ) ) ;
#3392=CARTESIAN_POINT ( 'NONE',  ( -13.57481594606304576, 33.21132812716787441, 5.622872871577880183 ) ) ;
#3397=CARTESIAN_POINT ( 'NONE',  ( 5.622872871577825116, 35.29492187716787299, -13.57481594606309372 ) ) ;
#3419=CARTESIAN_POINT ( 'NONE',  ( -13.14518615778179189, 33.65781250108393152, 5.444914386472304635 ) ) ;
#3448=ORIENTED_EDGE ( 'NONE', *, *, #12134, .T. ) ;
#3454=CARTESIAN_POINT ( 'NONE',  ( 13.14518615778179900, 32.26875000108393721, -5.444914386472297529 ) ) ;
#3466=CARTESIAN_POINT ( 'NONE',  ( -8.049105076161786076E-16, 35.59257812608393579, -13.14518615778179544 ) ) ;
#3479=ORIENTED_EDGE ( 'NONE', *, *, #1836, .F. ) ;
#3500=CONICAL_SURFACE ( 'NONE', #13019, 23.26794919243113213, 0.5235987755983000369 ) ;
#3503=DIRECTION ( 'NONE',  ( 0.000000000000000000, 0.000000000000000000, 1.000000000000000000 ) ) ;
#3504=CARTESIAN_POINT ( 'NONE',  ( 13.14518615778179544, 39.56132812608393579, -1.609821015232357215E-15 ) ) ;
#3515=CIRCLE ( 'NONE', #23529, 25.00000000000001066 ) ;
#3527=ADVANCED_FACE ( 'NONE', ( #5308 ), #17491, .T. ) ;
#3539=CARTESIAN_POINT ( 'NONE',  ( -11.69037824551319460, 35.99999999999998579, -6.307928093363390332 ) ) ;
#3540=CARTESIAN_POINT ( 'NONE',  ( -8.049105076161786076E-16, 31.82226562608393650, -13.14518615778179544 ) ) ;
#3541=CARTESIAN_POINT ( 'NONE',  ( 13.14518615778179722, 32.26875000108393721, -5.444914386472297529 ) ) ;
#3542=CARTESIAN_POINT ( 'NONE',  ( -9.598844408820454532, 31.67343750216787512, 9.598844408820459861 ) ) ;
#3563=CARTESIAN_POINT ( 'NONE',  ( -13.14518615778179900, 31.97109375108393436, -5.444914386472297529 ) ) ;
#3565=EDGE_CURVE ( 'NONE', #26666, #18529, #22067, .T. ) ;
#3583=CARTESIAN_POINT ( 'NONE',  ( -13.09590655363597733, 36.00000000000000000, 1.137167824541468031 ) ) ;
#3591=ORIENTED_EDGE ( 'NONE', *, *, #7284, .T. ) ;
#3596=VERTEX_POINT ( 'NONE', #22840 ) ;
#3598=CARTESIAN_POINT ( 'NONE',  ( -13.14518615778179544, 34.99726562608393721, 0.000000000000000000 ) ) ;
#3612=CARTESIAN_POINT ( 'NONE',  ( -8.049105076161786076E-16, 34.79882812608393294, -13.14518615778179544 ) ) ;
#3619=CARTESIAN_POINT ( 'NONE',  ( -8.312177448680279460E-16, 32.16953125216787157, -13.57481594606304576 ) ) ;
#3620=DIRECTION ( 'NONE',  ( 0.000000000000000000, 0.000000000000000000, 1.000000000000000000 ) ) ;
#3640=LINE ( 'NONE', #21302, #24379 ) ;
#3645=CARTESIAN_POINT ( 'NONE',  ( -13.14518615778179544, 39.16445312608393436, 0.000000000000000000 ) ) ;
#3652=ORIENTED_EDGE ( 'NONE', *, *, #24310, .F. ) ;
#3668=AXIS2_PLACEMENT_3D ( 'NONE', #15004, #23582, #19305 ) ;
#3679=CARTESIAN_POINT ( 'NONE',  ( -9.598844408820454532, 39.51171874999999289, 9.598844408820459861 ) ) ;
#3681=CARTESIAN_POINT ( 'NONE',  ( 5.622872871577878406, 32.61601562716786873, 13.57481594606304576 ) ) ;
#3705=CARTESIAN_POINT ( 'NONE',  ( -8.049105076161786076E-16, 32.61601562608393579, -13.14518615778179544 ) ) ;
#3735=CARTESIAN_POINT ( 'NONE',  ( 13.14518615778179544, 33.80664062608393294, -1.609821015232357215E-15 ) ) ;
#3745=EDGE_CURVE ( 'NONE', #13023, #12136, #16133, .T. ) ;
#3750=CARTESIAN_POINT ( 'NONE',  ( -5.444914386472299306, 33.55859375108393294, 13.14518615778179722 ) ) ;
#3764=EDGE_CURVE ( 'NONE', #19447, #15410, #17090, .T. ) ;
#3765=LINE ( 'NONE', #14155, #5523 ) ;
#3781=CARTESIAN_POINT ( 'NONE',  ( 5.622872871577878406, 34.20351562716788152, 13.57481594606304398 ) ) ;
#3785=FACE_OUTER_BOUND ( 'NONE', #12144, .T. ) ;
#3794=EDGE_CURVE ( 'NONE', #25494, #26327, #6565, .T. ) ;
#3800=PRESENTATION_STYLE_ASSIGNMENT (( #16485 ) ) ;
#3812=CARTESIAN_POINT ( 'NONE',  ( 9.598844408820456309, 40.70234374999999716, -9.598844408820458085 ) ) ;
#3813=CARTESIAN_POINT ( 'NONE',  ( 5.444914386472297529, 33.95546875108394147, -13.14518615778179722 ) ) ;
#3814=CARTESIAN_POINT ( 'NONE',  ( -8.312177448680279460E-16, 31.37578125216787583, -13.57481594606304576 ) ) ;
#3835=CARTESIAN_POINT ( 'NONE',  ( 5.444914386472302859, 34.65000000108393863, 13.14518615778179189 ) ) ;
#3842=CARTESIAN_POINT ( 'NONE',  ( 0.000000000000000000, 0.4999999999999970024, 0.000000000000000000 ) ) ;
#3867=CARTESIAN_POINT ( 'NONE',  ( -8.049105076161786076E-16, 35.79101562608394005, -13.14518615778179544 ) ) ;
#3868=CARTESIAN_POINT ( 'NONE',  ( 13.14518615778179544, 33.01289062608393010, -1.609821015232357215E-15 ) ) ;
#3871=CARTESIAN_POINT ( 'NONE',  ( -8.312177448680279460E-16, 31.37578125216787583, -13.57481594606304576 ) ) ;
#3875=EDGE_CURVE ( 'NONE', #25304, #12114, #13949, .T. ) ;
#3885=CARTESIAN_POINT ( 'NONE',  ( -8.049105076161786076E-16, 32.41757812608393863, -13.14518615778179544 ) ) ;
#3923=FACE_OUTER_BOUND ( 'NONE', #4866, .T. ) ;
#3924=AXIS2_PLACEMENT_3D ( 'NONE', #18616, #20896, #1378 ) ;
#3944=VECTOR ( 'NONE', #21325, 1000.000000000000000 ) ;
#3954=CARTESIAN_POINT ( 'NONE',  ( 13.57481594606304576, 40.60312499999999858, -1.662435489736055892E-15 ) ) ;
#3955=CARTESIAN_POINT ( 'NONE',  ( -5.444914386472297529, 31.67343750108393863, -13.14518615778179722 ) ) ;
#3957=CARTESIAN_POINT ( 'NONE',  ( 13.57481594606304931, 31.92148437716787512, 5.622872871577869525 ) ) ;
#3985=DIRECTION ( 'NONE',  ( -0.000000000000000000, -1.000000000000000000, -0.000000000000000000 ) ) ;
#3997=DIRECTION ( 'NONE',  ( -0.000000000000000000, -1.000000000000000000, -0.000000000000000000 ) ) ;
#4011=CARTESIAN_POINT ( 'NONE',  ( 13.14518615778179544, 34.60039062608392868, -1.609821015232357215E-15 ) ) ;
#4020=CARTESIAN_POINT ( 'NONE',  ( 0.000000000000000000, 0.4999999999999970024, 22.40192378864669465 ) ) ;
#4029=CARTESIAN_POINT ( 'NONE',  ( 3.755638265659908104, 31.58960998161716560, -13.14518615778179900 ) ) ;
#4040=VERTEX_POINT ( 'NONE', #17092 ) ;
#4044=CIRCLE ( 'NONE', #28108, 1.000000000000000888 ) ;
#4053=CARTESIAN_POINT ( 'NONE',  ( 2.493653234604083739E-15, 34.94765625216787441, 13.57481594606304576 ) ) ;
#4091=CARTESIAN_POINT ( 'NONE',  ( -5.444914386472297529, 32.46718750108393436, -13.14518615778179722 ) ) ;
#4094=CARTESIAN_POINT ( 'NONE',  ( -13.14518615778179544, 38.96601562608393721, 0.000000000000000000 ) ) ;
#4100=CARTESIAN_POINT ( 'NONE',  ( 0.000000000000000000, 36.00000000000000000, 0.000000000000000000 ) ) ;
#4124=CARTESIAN_POINT ( 'NONE',  ( 9.295050272127047819, 37.87460937608393863, 9.295050272127046043 ) ) ;
#4146=CARTESIAN_POINT ( 'NONE',  ( 13.57481594606304931, 32.61601562499999574, 5.622872871577868636 ) ) ;
#4147=EDGE_CURVE ( 'NONE', #11554, #25472, #19069, .T. ) ;
#4151=CARTESIAN_POINT ( 'NONE',  ( 13.14518615778179722, 35.54296875108394715, 5.444914386472293977 ) ) ;
#4152=CARTESIAN_POINT ( 'NONE',  ( -13.14518615778179900, 38.32109375108394289, -5.444914386472297529 ) ) ;
#4169=CARTESIAN_POINT ( 'NONE',  ( -9.295050272127046043, 33.31054687608393294, -9.295050272127046043 ) ) ;
#4173=CARTESIAN_POINT ( 'NONE',  ( 0.000000000000000000, 36.00000000000000000, 0.000000000000000000 ) ) ;
#4174=CARTESIAN_POINT ( 'NONE',  ( -13.09590655363597733, 36.00000000000000000, 1.137167824541468031 ) ) ;
#4181=ORIENTED_EDGE ( 'NONE', *, *, #4147, .F. ) ;
#4187=CARTESIAN_POINT ( 'NONE',  ( -5.622872871577782483, 34.60039062716787583, -13.57481594606313990 ) ) ;
#4210=AXIS2_PLACEMENT_3D ( 'NONE', #3842, #12373, #9966 ) ;
#4221=LINE ( 'NONE', #26307, #21882 ) ;
#4222=SURFACE_SIDE_STYLE ('',( #8212 ) ) ;
#4230=CARTESIAN_POINT ( 'NONE',  ( 13.14518615778179900, 37.72578125108393721, 5.444914386472293977 ) ) ;
#4246=CARTESIAN_POINT ( 'NONE',  ( 0.000000000000000000, 10.00000000000000178, 0.000000000000000000 ) ) ;
#4254=EDGE_LOOP ( 'NONE', ( #472, #20433, #20283, #6177 ) ) ;
#4257=CARTESIAN_POINT ( 'NONE',  ( -9.598844408820454532, 36.33671874999999574, 9.598844408820459861 ) ) ;
#4259=CARTESIAN_POINT ( 'NONE',  ( 2.414731522848535132E-15, 36.18789062608393436, 13.14518615778179544 ) ) ;
#4264=CARTESIAN_POINT ( 'NONE',  ( 0.000000000000000000, 36.00000000000000000, 0.000000000000000000 ) ) ;
#4266=EDGE_CURVE ( 'NONE', #19839, #18468, #23446, .T. ) ;
#4285=ORIENTED_EDGE ( 'NONE', *, *, #4299, .F. ) ;
#4287=CARTESIAN_POINT ( 'NONE',  ( -9.295050272127046043, 31.72304687608393081, -9.295050272127046043 ) ) ;
#4299=EDGE_CURVE ( 'NONE', #3596, #18166, #12148, .T. ) ;
#4308=CARTESIAN_POINT ( 'NONE',  ( 9.295050272127046043, 33.11210937608393579, -9.295050272127046043 ) ) ;
#4322=CARTESIAN_POINT ( 'NONE',  ( -13.14518615778179189, 39.80937500108392868, 5.444914386472304635 ) ) ;
#4325=( LENGTH_UNIT ( ) NAMED_UNIT ( * ) SI_UNIT ( .MILLI., .METRE. ) );
#4356=CARTESIAN_POINT ( 'NONE',  ( 2.493653234604083739E-15, 32.46718749999999432, 13.57481594606304576 ) ) ;
#4371=CARTESIAN_POINT ( 'NONE',  ( 5.444914386472302859, 40.00781250108393294, 13.14518615778179189 ) ) ;
#4401=CARTESIAN_POINT ( 'NONE',  ( 9.598844408820459861, 38.12265624999999858, 9.598844408820456309 ) ) ;
#4404=CARTESIAN_POINT ( 'NONE',  ( -5.444914386472297529, 36.63437500108393152, -13.14518615778179900 ) ) ;
#4417=ORIENTED_EDGE ( 'NONE', *, *, #7410, .T. ) ;
#4428=CARTESIAN_POINT ( 'NONE',  ( 2.849501950123402596E-15, 1.000000000000000000, -23.26794919243112858 ) ) ;
#4432=CARTESIAN_POINT ( 'NONE',  ( 9.295050272127047819, 33.90585937608393863, 9.295050272127046043 ) ) ;
#4433=CARTESIAN_POINT ( 'NONE',  ( 13.14518615778179544, 40.35507812608393863, -1.609821015232357215E-15 ) ) ;
#4436=CARTESIAN_POINT ( 'NONE',  ( 3.878384841496545388, 31.34156311272377238, -13.57481594606304753 ) ) ;
#4452=ORIENTED_EDGE ( 'NONE', *, *, #20813, .F. ) ;
#4473=ORIENTED_EDGE ( 'NONE', *, *, #1321, .T. ) ;
#4506=AXIS2_PLACEMENT_3D ( 'NONE', #13491, #13773, #11494 ) ;
#4512=CARTESIAN_POINT ( 'NONE',  ( -5.444914386472299306, 38.32109375108394289, 13.14518615778179722 ) ) ;
#4540=CARTESIAN_POINT ( 'NONE',  ( -9.598844408820454532, 37.92421874999999432, 9.598844408820459861 ) ) ;
#4541=CARTESIAN_POINT ( 'NONE',  ( 0.3745404134779373173, 36.00000000000003553, -13.51869779562201757 ) ) ;
#4542=CARTESIAN_POINT ( 'NONE',  ( 9.295050272127047819, 37.08085937608393579, 9.295050272127046043 ) ) ;
#4551=LINE ( 'NONE', #9626, #14531 ) ;
#4564=CARTESIAN_POINT ( 'NONE',  ( 13.57481594606304753, 32.81445312716787299, -5.622872871577873966 ) ) ;
#4568=CARTESIAN_POINT ( 'NONE',  ( -13.14518615778179900, 31.77265625108393365, -5.444914386472297529 ) ) ;
#4574=ORIENTED_EDGE ( 'NONE', *, *, #6386, .F. ) ;
#4601=CARTESIAN_POINT ( 'NONE',  ( 9.295050272127047819, 39.26367187608393294, 9.295050272127046043 ) ) ;
#4612=ORIENTED_EDGE ( 'NONE', *, *, #18222, .T. ) ;
#4640=CARTESIAN_POINT ( 'NONE',  ( 6.944426393311537993, 31.75150625057403175, -11.16113171639042356 ) ) ;
#4654=CARTESIAN_POINT ( 'NONE',  ( 13.14518615778179900, 37.82500000108392868, -5.444914386472297529 ) ) ;
#4666=VERTEX_POINT ( 'NONE', #16755 ) ;
#4674=CARTESIAN_POINT ( 'NONE',  ( 13.40642364673445819, 36.00000000000001421, 1.227293221035465454 ) ) ;
#4686=CARTESIAN_POINT ( 'NONE',  ( -8.312177448680279460E-16, 36.83281249999999574, -13.57481594606304576 ) ) ;
#4688=CARTESIAN_POINT ( 'NONE',  ( -9.295050272127044266, 38.46992187608393721, 9.295050272127047819 ) ) ;
#4696=ORIENTED_EDGE ( 'NONE', *, *, #20337, .T. ) ;
#4713=CARTESIAN_POINT ( 'NONE',  ( -8.049105076161786076E-16, 31.82226562608393650, -13.14518615778179544 ) ) ;
#4714=CARTESIAN_POINT ( 'NONE',  ( 13.14518615778179900, 38.81718750108393579, -5.444914386472297529 ) ) ;
#4745=ORIENTED_EDGE ( 'NONE', *, *, #2536, .F. ) ;
#4747=CARTESIAN_POINT ( 'NONE',  ( 13.14518615778179544, 38.56914062608393579, -1.609821015232357215E-15 ) ) ;
#4750=DIRECTION ( 'NONE',  ( -0.000000000000000000, -1.000000000000000000, -0.000000000000000000 ) ) ;
#4777=( BOUNDED_CURVE ( )  B_SPLINE_CURVE ( 2, ( #12305, #25574, #1509, #18745, #21161, #18873, #17007, #8043, #16601 ),
 .UNSPECIFIED., .F., .F. ) 
 B_SPLINE_CURVE_WITH_KNOTS ( ( 3, 2, 2, 2, 3 ),
 ( 0.6874999999999997780, 0.6979166666666665186, 0.7083333333333333703, 0.7187500000000001110, 0.7291666666666668517 ),
 .UNSPECIFIED. ) 
 CURVE ( )  GEOMETRIC_REPRESENTATION_ITEM ( )  RATIONAL_B_SPLINE_CURVE ( ( 1.000000000000001554, 0.9238795325112850731, 1.000000000000000000, 0.9238795325112867385, 1.000000000000000000, 0.9238795325112867385, 1.000000000000000000, 0.9238795325112850731, 1.000000000000001554 ) ) 
 REPRESENTATION_ITEM ( '' )  );
#4778=ORIENTED_EDGE ( 'NONE', *, *, #12329, .T. ) ;
#4797=CARTESIAN_POINT ( 'NONE',  ( 13.14518615778179900, 34.65000000108393152, -5.444914386472297529 ) ) ;
#4818=CARTESIAN_POINT ( 'NONE',  ( 7.065634988761035906, 35.99999999999999289, 11.21307450592191124 ) ) ;
#4823=CARTESIAN_POINT ( 'NONE',  ( -9.598844408820458085, 37.82500000216787583, -9.598844408820458085 ) ) ;
#4831=CYLINDRICAL_SURFACE ( 'NONE', #4506, 13.57481594606304576 ) ;
#4833=CARTESIAN_POINT ( 'NONE',  ( 9.598844408820459861, 36.53515624999999289, 9.598844408820456309 ) ) ;
#4835=CARTESIAN_POINT ( 'NONE',  ( 5.444914386472297529, 33.36015625108393579, -13.14518615778179900 ) ) ;
#4838=CARTESIAN_POINT ( 'NONE',  ( 5.622872871577878406, 36.58476562716787583, 13.57481594606304576 ) ) ;
#4857=ADVANCED_FACE ( 'NONE', ( #2365 ), #23885, .T. ) ;
#4859=CARTESIAN_POINT ( 'NONE',  ( 13.14518615778179544, 37.18007812608393436, -1.609821015232357215E-15 ) ) ;
#4862=ORIENTED_EDGE ( 'NONE', *, *, #6865, .F. ) ;
#4864=CARTESIAN_POINT ( 'NONE',  ( -13.57481594606304753, 32.21914062499999432, -5.622872871577872189 ) ) ;
#4866=EDGE_LOOP ( 'NONE', ( #20799, #4696, #17094, #281 ) ) ;
#4883=VECTOR ( 'NONE', #14865, 1000.000000000000114 ) ;
#4884=CARTESIAN_POINT ( 'NONE',  ( 0.000000000000000000, 36.00000000000000000, 0.000000000000000000 ) ) ;
#4892=CARTESIAN_POINT ( 'NONE',  ( -13.14518615778179900, 35.74140625108393721, -5.444914386472297529 ) ) ;
#4930=CARTESIAN_POINT ( 'NONE',  ( 2.354566838718444278E-15, 10.00000000000000000, -19.22649730810373470 ) ) ;
#4940=CARTESIAN_POINT ( 'NONE',  ( -5.444914386472297529, 34.84843750108393579, -13.14518615778179900 ) ) ;
#4952=CARTESIAN_POINT ( 'NONE',  ( 13.57481594606304576, 33.45937499999999432, -1.662435489736055892E-15 ) ) ;
#4966=CARTESIAN_POINT ( 'NONE',  ( -9.598844408820458085, 38.61875000216787157, -9.598844408820458085 ) ) ;
#4970=CARTESIAN_POINT ( 'NONE',  ( -13.57481594606304576, 33.16171875216787868, 0.000000000000000000 ) ) ;
#4973=CARTESIAN_POINT ( 'NONE',  ( -13.57481594606304576, 33.06249999999999289, 0.000000000000000000 ) ) ;
#4975=CARTESIAN_POINT ( 'NONE',  ( 13.14518615778179900, 35.54296875108394715, 5.444914386472293977 ) ) ;
#4977=CARTESIAN_POINT ( 'NONE',  ( 9.295050272127047819, 35.29492187608393294, 9.295050272127046043 ) ) ;
#4978=CARTESIAN_POINT ( 'NONE',  ( -5.622872871577873077, 35.39414062716787157, -13.57481594606304753 ) ) ;
#5001=FACE_OUTER_BOUND ( 'NONE', #18248, .T. ) ;
#5005=CARTESIAN_POINT ( 'NONE',  ( -13.14518615778179544, 36.78320312608393294, 0.000000000000000000 ) ) ;
#5012=CARTESIAN_POINT ( 'NONE',  ( -13.57481594606304753, 34.60039062499999574, -5.622872871577872189 ) ) ;
#5023=EDGE_LOOP ( 'NONE', ( #20899, #645, #28162, #17386 ) ) ;
#5033=CARTESIAN_POINT ( 'NONE',  ( 5.444914386472297529, 36.33671875108394289, -13.14518615778179900 ) ) ;
#5053=CARTESIAN_POINT ( 'NONE',  ( 2.493653234604083739E-15, 34.05468749999999289, 13.57481594606304576 ) ) ;
#5057=AXIS2_PLACEMENT_3D ( 'NONE', #25147, #10028, #12020 ) ;
#5081=CARTESIAN_POINT ( 'NONE',  ( 2.414731522848535132E-15, 35.19570312608392726, 13.14518615778179544 ) ) ;
#5103=CARTESIAN_POINT ( 'NONE',  ( -8.312177448680279460E-16, 40.10703125216787157, -13.57481594606304576 ) ) ;
#5106=CARTESIAN_POINT ( 'NONE',  ( -9.598844408820454532, 33.26093750216787726, 9.598844408820459861 ) ) ;
#5109=CARTESIAN_POINT ( 'NONE',  ( -8.312177448680279460E-16, 35.24531249999999716, -13.57481594606304576 ) ) ;
#5110=CARTESIAN_POINT ( 'NONE',  ( -5.622872871577873077, 32.91367187499999858, -13.57481594606304753 ) ) ;
#5112=CARTESIAN_POINT ( 'NONE',  ( -5.444914386472299306, 35.34453125108393579, 13.14518615778179722 ) ) ;
#5114=CARTESIAN_POINT ( 'NONE',  ( -13.14518615778179189, 35.04687500108393294, 5.444914386472304635 ) ) ;
#5115=CARTESIAN_POINT ( 'NONE',  ( -13.57481594606304753, 37.08085937716786873, -5.622872871577873077 ) ) ;
#5139=CARTESIAN_POINT ( 'NONE',  ( -13.14518615778179900, 35.93984375108393436, -5.444914386472297529 ) ) ;
#5150=DIRECTION ( 'NONE',  ( 0.000000000000000000, 0.000000000000000000, -1.000000000000000000 ) ) ;
#5173=CARTESIAN_POINT ( 'NONE',  ( -5.444914386472299306, 37.52734375108393294, 13.14518615778179722 ) ) ;
#5180=EDGE_CURVE ( 'NONE', #5426, #15725, #17035, .T. ) ;
#5197=ORIENTED_EDGE ( 'NONE', *, *, #27168, .T. ) ;
#5222=CARTESIAN_POINT ( 'NONE',  ( 0.000000000000000000, 23.00000000000000000, 0.000000000000000000 ) ) ;
#5251=CYLINDRICAL_SURFACE ( 'NONE', #19521, 23.00000000000001421 ) ;
#5253=CARTESIAN_POINT ( 'NONE',  ( 5.622872871577871301, 33.60820312499998863, -13.57481594606304753 ) ) ;
#5255=CARTESIAN_POINT ( 'NONE',  ( -13.14518615778179544, 32.81445312608393294, 0.000000000000000000 ) ) ;
#5257=CARTESIAN_POINT ( 'NONE',  ( -5.444914386472297529, 34.84843750108393579, -13.14518615778179722 ) ) ;
#5258=CARTESIAN_POINT ( 'NONE',  ( 2.493653234604083739E-15, 37.32890625216786873, 13.57481594606304576 ) ) ;
#5283=CARTESIAN_POINT ( 'NONE',  ( 13.14518615778179544, 34.79882812608394005, -1.609821015232357215E-15 ) ) ;
#5305=DIRECTION ( 'NONE',  ( 0.000000000000000000, 0.000000000000000000, 1.000000000000000000 ) ) ;
#5308=FACE_OUTER_BOUND ( 'NONE', #1978, .T. ) ;
#5316=CARTESIAN_POINT ( 'NONE',  ( -9.295050272127044266, 35.09648437608392868, 9.295050272127047819 ) ) ;
#5353=EDGE_CURVE ( 'NONE', #20971, #22337, #12113, .T. ) ;
#5369=AXIS2_PLACEMENT_3D ( 'NONE', #13301, #17455, #11028 ) ;
#5388=CARTESIAN_POINT ( 'NONE',  ( -5.622872871577873077, 38.07304687716787583, 13.57481594606304753 ) ) ;
#5397=CARTESIAN_POINT ( 'NONE',  ( -13.57481594606304576, 33.90585937500000568, 5.622872871577880183 ) ) ;
#5398=CARTESIAN_POINT ( 'NONE',  ( -12.85950995607747949, 36.00000000000000711, -3.245221471867173246 ) ) ;
#5399=CARTESIAN_POINT ( 'NONE',  ( -5.444914386472297529, 34.25312500108393010, -13.14518615778179900 ) ) ;
#5402=CARTESIAN_POINT ( 'NONE',  ( 2.493653234604083739E-15, 35.74140625216787015, 13.57481594606304576 ) ) ;
#5416=CARTESIAN_POINT ( 'NONE',  ( 1.662435489736055892E-15, 36.00000000000000000, 13.57481594606304576 ) ) ;
#5426=VERTEX_POINT ( 'NONE', #7652 ) ;
#5427=CARTESIAN_POINT ( 'NONE',  ( -13.14518615778179544, 37.57695312608393579, 0.000000000000000000 ) ) ;
#5448=FACE_OUTER_BOUND ( 'NONE', #6321, .T. ) ;
#5457=CARTESIAN_POINT ( 'NONE',  ( 9.295050272127047819, 37.67617187608393436, 9.295050272127046043 ) ) ;
#5496=FACE_OUTER_BOUND ( 'NONE', #10822, .T. ) ;
#5510=CARTESIAN_POINT ( 'NONE',  ( -9.295050272127044266, 39.26367187608393294, 9.295050272127047819 ) ) ;
#5511=CARTESIAN_POINT ( 'NONE',  ( 2.849501950123402202E-15, 1.000000000000000000, -23.26794919243112503 ) ) ;
#5517=CARTESIAN_POINT ( 'NONE',  ( 2.849501950123402596E-15, 0.000000000000000000, -23.26794919243112858 ) ) ;
#5523=VECTOR ( 'NONE', #20594, 1000.000000000000000 ) ;
#5526=CARTESIAN_POINT ( 'NONE',  ( 13.14518615778179544, 33.21132812608393436, -1.609821015232357215E-15 ) ) ;
#5528=ADVANCED_FACE ( 'NONE', ( #18851 ), #27559, .T. ) ;
#5531=ORIENTED_EDGE ( 'NONE', *, *, #20675, .T. ) ;
#5532=SURFACE_SIDE_STYLE ('',( #6455 ) ) ;
#5541=CARTESIAN_POINT ( 'NONE',  ( -13.57481594606304576, 34.64999999999999147, 0.000000000000000000 ) ) ;
#5544=CARTESIAN_POINT ( 'NONE',  ( -13.57481594606304576, 40.25585937499999289, 5.622872871577880183 ) ) ;
#5546=CARTESIAN_POINT ( 'NONE',  ( -13.14518615778179722, 35.74140625108393721, -5.444914386472297529 ) ) ;
#5548=CARTESIAN_POINT ( 'NONE',  ( 13.57481594606304931, 34.30273437716787299, 5.622872871577869525 ) ) ;
#5559=EDGE_LOOP ( 'NONE', ( #27877, #9683, #2537, #23662 ) ) ;
#5571=CARTESIAN_POINT ( 'NONE',  ( 13.14518615778179900, 33.95546875108393436, 5.444914386472293977 ) ) ;
#5573=CARTESIAN_POINT ( 'NONE',  ( 2.493653234604083739E-15, 35.74140625216787015, 13.57481594606304576 ) ) ;
#5576=CARTESIAN_POINT ( 'NONE',  ( 3.061616997868383831E-15, 20.00000000000000000, -25.00000000000000711 ) ) ;
#5600=CARTESIAN_POINT ( 'NONE',  ( -13.14518615778179900, 32.56640625108394005, -5.444914386472297529 ) ) ;
#5612=CARTESIAN_POINT ( 'NONE',  ( -5.444914386472299306, 36.73359375108393010, 13.14518615778179722 ) ) ;
#5645=CARTESIAN_POINT ( 'NONE',  ( 13.57481594606304576, 34.35234375216787583, -1.662435489736055892E-15 ) ) ;
#5647=CARTESIAN_POINT ( 'NONE',  ( 0.000000000000000000, 36.00000000000000000, -11.57481594606304576 ) ) ;
#5648=CARTESIAN_POINT ( 'NONE',  ( 9.295050272127046043, 40.45429687608393721, -9.295050272127046043 ) ) ;
#5650=CARTESIAN_POINT ( 'NONE',  ( 0.000000000000000000, 1.000000000000000000, 0.000000000000000000 ) ) ;
#5654=CARTESIAN_POINT ( 'NONE',  ( -8.312177448680279460E-16, 32.07031249999999289, -13.57481594606304576 ) ) ;
#5668=CARTESIAN_POINT ( 'NONE',  ( -9.598844408820454532, 33.95546874999999432, 9.598844408820459861 ) ) ;
#5677=CARTESIAN_POINT ( 'NONE',  ( -9.598844408820454532, 32.36796874999999574, 9.598844408820459861 ) ) ;
#5680=CARTESIAN_POINT ( 'NONE',  ( -13.57481594606304576, 39.46210937499999005, 5.622872871577880183 ) ) ;
#5682=CARTESIAN_POINT ( 'NONE',  ( -9.295050272127046043, 31.72304687608393081, -9.295050272127046043 ) ) ;
#5683=CARTESIAN_POINT ( 'NONE',  ( -13.57481594606304576, 32.41757812716787157, 5.622872871577880183 ) ) ;
#5696=FACE_OUTER_BOUND ( 'NONE', #1107, .T. ) ;
#5704=ADVANCED_FACE ( 'NONE', ( #2459 ), #24395, .T. ) ;
#5708=CARTESIAN_POINT ( 'NONE',  ( 13.14518615778179900, 32.36796875108393579, 5.444914386472293977 ) ) ;
#5726=CARTESIAN_POINT ( 'NONE',  ( -0.5932557025495835967, 36.00000000000000000, 13.13889047851777292 ) ) ;
#5731=AXIS2_PLACEMENT_3D ( 'NONE', #15828, #24817, #13821 ) ;
#5739=CARTESIAN_POINT ( 'NONE',  ( -9.295050272127046043, 32.51679687608393721, -9.295050272127046043 ) ) ;
#5752=CARTESIAN_POINT ( 'NONE',  ( -13.14518615778179900, 34.94765625108392726, -5.444914386472297529 ) ) ;
#5776=EDGE_CURVE ( 'NONE', #12136, #19447, #13547, .T. ) ;
#5782=CIRCLE ( 'NONE', #16701, 19.22649730810373470 ) ;
#5786=CARTESIAN_POINT ( 'NONE',  ( -5.444914386472299306, 39.31328125108394289, 13.14518615778179722 ) ) ;
#5817=CARTESIAN_POINT ( 'NONE',  ( -9.598844408820454532, 40.30546874999999574, 9.598844408820459861 ) ) ;
#5819=CARTESIAN_POINT ( 'NONE',  ( 5.622872871577878406, 33.40976562716787157, 13.57481594606304576 ) ) ;
#5842=CARTESIAN_POINT ( 'NONE',  ( -13.14518615778179900, 34.35234375108393579, -5.444914386472297529 ) ) ;
#5865=ORIENTED_EDGE ( 'NONE', *, *, #27798, .T. ) ;
#5871=ORIENTED_EDGE ( 'NONE', *, *, #25176, .T. ) ;
#5876=CARTESIAN_POINT ( 'NONE',  ( -5.444914386472297529, 34.84843750108393579, -13.14518615778179900 ) ) ;
#5883=EDGE_LOOP ( 'NONE', ( #12035, #24685 ) ) ;
#5892=CARTESIAN_POINT ( 'NONE',  ( 5.444914386472302859, 33.65781250108393152, 13.14518615778179189 ) ) ;
#5905=ORIENTED_EDGE ( 'NONE', *, *, #9151, .T. ) ;
#5918=ORIENTED_EDGE ( 'NONE', *, *, #12134, .F. ) ;
#5923=CARTESIAN_POINT ( 'NONE',  ( 9.598844408820456309, 34.45156250216787441, -9.598844408820458085 ) ) ;
#5929=ORIENTED_EDGE ( 'NONE', *, *, #27798, .F. ) ;
#5953=CARTESIAN_POINT ( 'NONE',  ( 9.598844408820459861, 38.91640624999999432, 9.598844408820456309 ) ) ;
#5955=CARTESIAN_POINT ( 'NONE',  ( 13.57481594606304753, 32.02070312716787015, -5.622872871577873077 ) ) ;
#5981=CARTESIAN_POINT ( 'NONE',  ( 4.157286354961724939, 36.00000000000000000, -12.92256159328856135 ) ) ;
#5983=CARTESIAN_POINT ( 'NONE',  ( 0.000000000000000000, 36.00000000000000000, 0.000000000000000000 ) ) ;
#5995=CARTESIAN_POINT ( 'NONE',  ( -11.26481880218173615, 35.99999999999999289, 6.828991891054706720 ) ) ;
#6000=EDGE_CURVE ( 'NONE', #4040, #15812, #8386, .T. ) ;
#6001=CARTESIAN_POINT ( 'NONE',  ( -8.312177448680279460E-16, 31.37578125216787583, -13.57481594606304576 ) ) ;
#6010=CARTESIAN_POINT ( 'NONE',  ( -5.444914386472297529, 34.05468750108393294, -13.14518615778179900 ) ) ;
#6027=CARTESIAN_POINT ( 'NONE',  ( -13.14518615778179544, 33.40976562608393863, 0.000000000000000000 ) ) ;
#6033=DIRECTION ( 'NONE',  ( -0.000000000000000000, -1.000000000000000000, -0.000000000000000000 ) ) ;
#6043=DIRECTION ( 'NONE',  ( 0.000000000000000000, 0.000000000000000000, 1.000000000000000000 ) ) ;
#6048=CIRCLE ( 'NONE', #4210, 22.40192378864669109 ) ;
#6058=CARTESIAN_POINT ( 'NONE',  ( 1.662435489736055892E-15, 36.00000000000000000, 13.57481594606304576 ) ) ;
#6063=DIRECTION ( 'NONE',  ( 0.000000000000000000, 0.000000000000000000, 1.000000000000000000 ) ) ;
#6087=CYLINDRICAL_SURFACE ( 'NONE', #10241, 13.57481594606304576 ) ;
#6088=CARTESIAN_POINT ( 'NONE',  ( -5.622872871577873077, 40.85117187499999147, -13.57481594606304753 ) ) ;
#6089=CARTESIAN_POINT ( 'NONE',  ( -9.295050272127044266, 31.92148437608393508, 9.295050272127047819 ) ) ;
#6090=CARTESIAN_POINT ( 'NONE',  ( 9.598844408820459861, 33.45937500216787441, 9.598844408820456309 ) ) ;
#6114=CARTESIAN_POINT ( 'NONE',  ( 13.57481594606304931, 35.89023437716787868, 5.622872871577868636 ) ) ;
#6117=DIRECTION ( 'NONE',  ( 0.000000000000000000, 0.000000000000000000, 1.000000000000000000 ) ) ;
#6130=CARTESIAN_POINT ( 'NONE',  ( -2.117096883972749467E-15, 29.95886589889650509, -11.57481594606304576 ) ) ;
#6144=CARTESIAN_POINT ( 'NONE',  ( 13.14518615778179544, 34.79882812608394005, -1.609821015232357215E-15 ) ) ;
#6145=CARTESIAN_POINT ( 'NONE',  ( 9.295050272127046043, 32.31835937608393294, -9.295050272127046043 ) ) ;
#6162=CARTESIAN_POINT ( 'NONE',  ( -13.14518615778179189, 32.66562500108393863, 5.444914386472304635 ) ) ;
#6177=ORIENTED_EDGE ( 'NONE', *, *, #17078, .F. ) ;
#6180=VECTOR ( 'NONE', #3997, 1000.000000000000000 ) ;
#6191=DIRECTION ( 'NONE',  ( -1.003171929053526103E-16, -0.5735764363510443831, -0.8191520442889929088 ) ) ;
#6225=ORIENTED_EDGE ( 'NONE', *, *, #5776, .F. ) ;
#6228=CARTESIAN_POINT ( 'NONE',  ( -13.14518615778179189, 33.45937500108393436, 5.444914386472304635 ) ) ;
#6229=CARTESIAN_POINT ( 'NONE',  ( -9.295050272127044266, 39.06523437608392868, 9.295050272127047819 ) ) ;
#6249=VECTOR ( 'NONE', #22171, 1000.000000000000000 ) ;
#6264=CARTESIAN_POINT ( 'NONE',  ( -12.99948823019059319, 35.99999999999999289, 1.999176114741941346 ) ) ;
#6276=EDGE_CURVE ( 'NONE', #25525, #20971, #22153, .T. ) ;
#6278=CARTESIAN_POINT ( 'NONE',  ( 9.295050272127046043, 34.89804687608393863, -9.295050272127046043 ) ) ;
#6279=CARTESIAN_POINT ( 'NONE',  ( 5.444914386472297529, 38.12265625108393152, -13.14518615778179900 ) ) ;
#6296=CARTESIAN_POINT ( 'NONE',  ( 13.14518615778179900, 32.96328125108393436, 5.444914386472293977 ) ) ;
#6307=ORIENTED_EDGE ( 'NONE', *, *, #12599, .T. ) ;
#6318=CARTESIAN_POINT ( 'NONE',  ( -8.312177448680279460E-16, 35.34453125216787583, -13.57481594606304576 ) ) ;
#6321=EDGE_LOOP ( 'NONE', ( #8543, #3591, #244, #10437 ) ) ;
#6357=ORIENTED_EDGE ( 'NONE', *, *, #13284, .F. ) ;
#6363=CARTESIAN_POINT ( 'NONE',  ( 9.295050272127046043, 39.46210937608393010, -9.295050272127046043 ) ) ;
#6381=DIRECTION ( 'NONE',  ( 0.000000000000000000, 1.000000000000000000, 0.000000000000000000 ) ) ;
#6386=EDGE_CURVE ( 'NONE', #9781, #10399, #8182, .T. ) ;
#6396=CARTESIAN_POINT ( 'NONE',  ( 13.14518615778179900, 36.43593750108392726, -5.444914386472297529 ) ) ;
#6420=CARTESIAN_POINT ( 'NONE',  ( -9.295050272127046043, 35.09648437608393579, -9.295050272127046043 ) ) ;
#6421=CARTESIAN_POINT ( 'NONE',  ( 9.295050272127047819, 40.25585937608393294, 9.295050272127046043 ) ) ;
#6436=CARTESIAN_POINT ( 'NONE',  ( 0.000000000000000000, 36.00000000000000000, 0.000000000000000000 ) ) ;
#6438=CARTESIAN_POINT ( 'NONE',  ( 9.295050272127047819, 33.70742187608393436, 9.295050272127046043 ) ) ;
#6441=ORIENTED_EDGE ( 'NONE', *, *, #18222, .F. ) ;
#6452=CARTESIAN_POINT ( 'NONE',  ( 2.414731522848535132E-15, 38.37070312608393152, 13.14518615778179544 ) ) ;
#6455=SURFACE_STYLE_FILL_AREA ( #25318 ) ;
#6457=CARTESIAN_POINT ( 'NONE',  ( -9.598844408820458085, 34.65000000216787868, -9.598844408820458085 ) ) ;
#6459=ORIENTED_EDGE ( 'NONE', *, *, #12876, .F. ) ;
#6481=DIRECTION ( 'NONE',  ( 0.000000000000000000, 1.000000000000000000, 0.000000000000000000 ) ) ;
#6484=LINE ( 'NONE', #27881, #3944 ) ;
#6485=CARTESIAN_POINT ( 'NONE',  ( 13.14518615778179900, 33.16171875108393863, 5.444914386472293977 ) ) ;
#6490=DIRECTION ( 'NONE',  ( -0.000000000000000000, -1.000000000000000000, -0.000000000000000000 ) ) ;
#6497=CARTESIAN_POINT ( 'NONE',  ( -9.295050272127044266, 39.85898437608393152, 9.295050272127047819 ) ) ;
#6504=ADVANCED_FACE ( 'NONE', ( #8354 ), #6087, .T. ) ;
#6505=DIRECTION ( 'NONE',  ( 0.000000000000000000, 0.000000000000000000, -1.000000000000000000 ) ) ;
#6525=CARTESIAN_POINT ( 'NONE',  ( -5.622872871577873077, 37.67617187499999432, -13.57481594606304753 ) ) ;
#6527=CARTESIAN_POINT ( 'NONE',  ( -13.14518615778179189, 36.83281250108393579, 5.444914386472304635 ) ) ;
#6537=CARTESIAN_POINT ( 'NONE',  ( 0.000000000000000000, 10.00000000000000000, 19.22649730810373470 ) ) ;
#6552=CARTESIAN_POINT ( 'NONE',  ( 13.14518615778179722, 33.95546875108394147, 5.444914386472293977 ) ) ;
#6553=CARTESIAN_POINT ( 'NONE',  ( -5.444914386472299306, 40.10703125108393152, 13.14518615778179722 ) ) ;
#6565=CIRCLE ( 'NONE', #25675, 23.00000000000001421 ) ;
#6596=ORIENTED_EDGE ( 'NONE', *, *, #6276, .T. ) ;
#6608=ORIENTED_EDGE ( 'NONE', *, *, #6865, .T. ) ;
#6611=COLOUR_RGB ( '', 0.40784314, 0.44705882, 0.49803922) ;
#6635=CARTESIAN_POINT ( 'NONE',  ( 5.444914386472302859, 38.42031250108393436, 13.14518615778179189 ) ) ;
#6662=CARTESIAN_POINT ( 'NONE',  ( -13.57481594606304753, 32.31835937716787299, -5.622872871577872189 ) ) ;
#6663=CARTESIAN_POINT ( 'NONE',  ( 5.622872871577878406, 38.86679687499999858, 13.57481594606304576 ) ) ;
#6665=CARTESIAN_POINT ( 'NONE',  ( -9.295050272127046043, 39.06523437608392868, -9.295050272127046043 ) ) ;
#6682=EDGE_CURVE ( 'NONE', #15854, #12047, #19837, .T. ) ;
#6689=CARTESIAN_POINT ( 'NONE',  ( -8.049105076161786076E-16, 31.62382812608393579, -13.14518615778179544 ) ) ;
#6701=EDGE_CURVE ( 'NONE', #19839, #21429, #23027, .T. ) ;
#6726=CARTESIAN_POINT ( 'NONE',  ( -9.295050272127046043, 38.86679687608393863, -9.295050272127046043 ) ) ;
#6728=VECTOR ( 'NONE', #22651, 1000.000000000000000 ) ;
#6776=AXIS2_PLACEMENT_3D ( 'NONE', #7774, #14033, #3503 ) ;
#6777=CARTESIAN_POINT ( 'NONE',  ( 5.444914386472297529, 37.92421875108392726, -13.14518615778179900 ) ) ;
#6787=ORIENTED_EDGE ( 'NONE', *, *, #7622, .T. ) ;
#6794=CARTESIAN_POINT ( 'NONE',  ( 12.00957333851164854, 36.00000000000000000, 5.901833544881618820 ) ) ;
#6807=CARTESIAN_POINT ( 'NONE',  ( -5.622872871577873077, 37.18007812500000853, 13.57481594606304753 ) ) ;
#6808=CARTESIAN_POINT ( 'NONE',  ( -1.816500417285228597, 36.00000000000000711, -13.35830014193482285 ) ) ;
#6809=CARTESIAN_POINT ( 'NONE',  ( 5.444914386472302859, 38.61875000108393152, 13.14518615778179189 ) ) ;
#6831=DIRECTION ( 'NONE',  ( 0.000000000000000000, 1.000000000000000000, 0.000000000000000000 ) ) ;
#6834=CARTESIAN_POINT ( 'NONE',  ( 5.444914386472302859, 33.85625000108393579, 13.14518615778179189 ) ) ;
#6835=CARTESIAN_POINT ( 'NONE',  ( 13.14518615778179900, 40.40468750108393436, -5.444914386472297529 ) ) ;
#6865=EDGE_CURVE ( 'NONE', #19382, #22143, #3640, .T. ) ;
#6871=CARTESIAN_POINT ( 'NONE',  ( -5.444914386472297529, 40.40468750108393436, -13.14518615778179900 ) ) ;
#6872=CARTESIAN_POINT ( 'NONE',  ( 0.000000000000000000, 20.00000000000000000, 25.00000000000000711 ) ) ;
#6881=ORIENTED_EDGE ( 'NONE', *, *, #3086, .T. ) ;
#6894=ORIENTED_EDGE ( 'NONE', *, *, #27480, .T. ) ;
#6907=ADVANCED_FACE ( 'NONE', ( #8854 ), #2028, .T. ) ;
#6916=CARTESIAN_POINT ( 'NONE',  ( -5.444914386472297529, 36.43593750108392726, -13.14518615778179900 ) ) ;
#6940=CARTESIAN_POINT ( 'NONE',  ( -13.57481594606304753, 37.87460937716787868, -5.622872871577873077 ) ) ;
#6949=CARTESIAN_POINT ( 'NONE',  ( 5.622872871577871301, 37.57695312499998863, -13.57481594606304753 ) ) ;
#6951=CARTESIAN_POINT ( 'NONE',  ( 2.414731522848535132E-15, 33.80664062608393294, 13.14518615778179544 ) ) ;
#6969=CIRCLE ( 'NONE', #12404, 11.57481594606304576 ) ;
#6976=CARTESIAN_POINT ( 'NONE',  ( -13.14518615778179189, 36.83281250108393579, 5.444914386472304635 ) ) ;
#6979=CARTESIAN_POINT ( 'NONE',  ( -9.598844408820458085, 32.16953124999999147, -9.598844408820458085 ) ) ;
#6997=VERTEX_POINT ( 'NONE', #8999 ) ;
#7007=CARTESIAN_POINT ( 'NONE',  ( -13.14518615778179189, 37.42812500108393436, 5.444914386472304635 ) ) ;
#7010=CARTESIAN_POINT ( 'NONE',  ( 0.000000000000000000, 23.00000000000000000, -23.00000000000001421 ) ) ;
#7039=LINE ( 'NONE', #2370, #6249 ) ;
#7052=CARTESIAN_POINT ( 'NONE',  ( 9.295050272127047819, 36.08867187608392868, 9.295050272127046043 ) ) ;
#7058=STYLED_ITEM ( 'NONE', ( #3800 ), #16871 ) ;
#7078=CARTESIAN_POINT ( 'NONE',  ( 9.598844408820459861, 39.01562500216787299, 9.598844408820456309 ) ) ;
#7082=CARTESIAN_POINT ( 'NONE',  ( 0.000000000000000000, 23.00000000000000000, 0.000000000000000000 ) ) ;
#7085=CARTESIAN_POINT ( 'NONE',  ( -13.57481594606304753, 33.80664062500000000, -5.622872871577873077 ) ) ;
#7087=CARTESIAN_POINT ( 'NONE',  ( -13.14518615778179189, 32.86406250108393579, 5.444914386472304635 ) ) ;
#7091=CARTESIAN_POINT ( 'NONE',  ( -5.622872871577873077, 36.48554687716787015, 13.57481594606304753 ) ) ;
#7109=ORIENTED_EDGE ( 'NONE', *, *, #17152, .F. ) ;
#7113=CARTESIAN_POINT ( 'NONE',  ( 2.414731522848535132E-15, 37.77539062608393294, 13.14518615778179544 ) ) ;
#7147=CARTESIAN_POINT ( 'NONE',  ( 13.14518615778179900, 36.13828125108393863, 5.444914386472293977 ) ) ;
#7158=EDGE_LOOP ( 'NONE', ( #13000, #16890, #7733, #19744 ) ) ;
#7190=CARTESIAN_POINT ( 'NONE',  ( -9.295050272127046043, 37.27929687608393294, -9.295050272127046043 ) ) ;
#7202=CARTESIAN_POINT ( 'NONE',  ( 2.493653234604083739E-15, 33.26093749999999716, 13.57481594606304576 ) ) ;
#7217=CARTESIAN_POINT ( 'NONE',  ( -5.622872871577873077, 38.86679687716788578, 13.57481594606304753 ) ) ;
#7223=CYLINDRICAL_SURFACE ( 'NONE', #7298, 11.57481594606304576 ) ;
#7227=CARTESIAN_POINT ( 'NONE',  ( -8.312177448680279460E-16, 33.65781249999999147, -13.57481594606304576 ) ) ;
#7229=CARTESIAN_POINT ( 'NONE',  ( 9.295050272127046043, 35.69179687608394147, -9.295050272127046043 ) ) ;
#7231=CARTESIAN_POINT ( 'NONE',  ( 1.137167824541903460, 36.00000000000000000, 13.09590655363594180 ) ) ;
#7232=CARTESIAN_POINT ( 'NONE',  ( 9.598844408820459861, 36.63437500216787157, 9.598844408820456309 ) ) ;
#7259=CARTESIAN_POINT ( 'NONE',  ( 9.295050272127047819, 35.49335937608393721, 9.295050272127046043 ) ) ;
#7265=( BOUNDED_CURVE ( )  B_SPLINE_CURVE ( 2, ( #22338, #2943, #13468, #2529, #4952, #24325, #17770, #2808, #7202 ),
 .UNSPECIFIED., .F., .F. ) 
 B_SPLINE_CURVE_WITH_KNOTS ( ( 3, 2, 2, 2, 3 ),
 ( 0.7708333333333333703, 0.7812500000000000000, 0.7916666666666665186, 0.8020833333333332593, 0.8124999999999998890 ),
 .UNSPECIFIED. ) 
 CURVE ( )  GEOMETRIC_REPRESENTATION_ITEM ( )  RATIONAL_B_SPLINE_CURVE ( ( 1.000000000000000000, 0.9238795325112867385, 1.000000000000000000, 0.9238795325112867385, 1.000000000000000000, 0.9238795325112867385, 1.000000000000000000, 0.9238795325112875156, 0.9999999999999992228 ) ) 
 REPRESENTATION_ITEM ( '' )  );
#7282=DIRECTION ( 'NONE',  ( 0.000000000000000000, 1.000000000000000000, 0.000000000000000000 ) ) ;
#7284=EDGE_CURVE ( 'NONE', #15725, #4666, #4551, .T. ) ;
#7292=CARTESIAN_POINT ( 'NONE',  ( 5.444914386472297529, 37.92421875108392726, -13.14518615778179900 ) ) ;
#7298=AXIS2_PLACEMENT_3D ( 'NONE', #27207, #20207, #27062 ) ;
#7300=( BOUNDED_CURVE ( )  B_SPLINE_CURVE ( 2, ( #15064, #2551, #12917, #13345, #26197, #6662, #24205, #11072, #19927 ),
 .UNSPECIFIED., .F., .F. ) 
 B_SPLINE_CURVE_WITH_KNOTS ( ( 3, 2, 2, 2, 3 ),
 ( 0.8124999999999998890, 0.8229166666666666297, 0.8333333333333334814, 0.8437500000000003331, 0.8541666666666670737 ),
 .UNSPECIFIED. ) 
 CURVE ( )  GEOMETRIC_REPRESENTATION_ITEM ( )  RATIONAL_B_SPLINE_CURVE ( ( 1.000000000000000888, 0.9238795325112859613, 1.000000000000000000, 0.9238795325112867385, 1.000000000000000000, 0.9238795325112867385, 1.000000000000000000, 0.9238795325112835188, 1.000000000000003331 ) ) 
 REPRESENTATION_ITEM ( '' )  );
#7338=FACE_OUTER_BOUND ( 'NONE', #5023, .T. ) ;
#7339=CARTESIAN_POINT ( 'NONE',  ( 13.14518615778179544, 36.18789062608393436, -1.609821015232357215E-15 ) ) ;
#7358=CARTESIAN_POINT ( 'NONE',  ( -13.14518615778179544, 33.60820312608393579, 0.000000000000000000 ) ) ;
#7361=CARTESIAN_POINT ( 'NONE',  ( -13.57481594606304753, 38.66835937716786731, -5.622872871577873077 ) ) ;
#7369=CARTESIAN_POINT ( 'NONE',  ( -5.622872871577873077, 35.59257812499999574, 13.57481594606304753 ) ) ;
#7370=CARTESIAN_POINT ( 'NONE',  ( -4.972887739508807137, 36.00000000000002842, -12.48139679469879582 ) ) ;
#7371=CARTESIAN_POINT ( 'NONE',  ( -5.444914386472297529, 33.45937500108394147, -13.14518615778179900 ) ) ;
#7374=CARTESIAN_POINT ( 'NONE',  ( -5.444914386472299306, 35.93984375108392726, 13.14518615778179722 ) ) ;
#7375=CARTESIAN_POINT ( 'NONE',  ( 2.493653234604083739E-15, 36.53515625216787299, 13.57481594606304576 ) ) ;
#7400=CARTESIAN_POINT ( 'NONE',  ( 9.295050272127046043, 36.48554687608393721, -9.295050272127046043 ) ) ;
#7404=DIRECTION ( 'NONE',  ( 0.000000000000000000, 0.000000000000000000, 1.000000000000000000 ) ) ;
#7410=EDGE_CURVE ( 'NONE', #21904, #19382, #27318, .T. ) ;
#7420=EDGE_CURVE ( 'NONE', #3329, #21904, #909, .T. ) ;
#7432=CARTESIAN_POINT ( 'NONE',  ( -5.444914386472299306, 36.73359375108393010, 13.14518615778179722 ) ) ;
#7482=FACE_OUTER_BOUND ( 'NONE', #25796, .T. ) ;
#7486=DIRECTION ( 'NONE',  ( 1.000000000000000000, -0.000000000000000000, 1.224646799147353207E-16 ) ) ;
#7492=EDGE_LOOP ( 'NONE', ( #6441, #13510, #21444, #25657 ) ) ;
#7504=CARTESIAN_POINT ( 'NONE',  ( 6.944426393311537993, 31.75150625057403175, -11.16113171639042356 ) ) ;
#7508=CARTESIAN_POINT ( 'NONE',  ( 9.598844408820459861, 38.22187500216787015, 9.598844408820456309 ) ) ;
#7517=CARTESIAN_POINT ( 'NONE',  ( 9.598844408820459861, 34.94765624999999432, 9.598844408820456309 ) ) ;
#7519=CARTESIAN_POINT ( 'NONE',  ( 13.14518615778179900, 35.64218750108393152, -5.444914386472297529 ) ) ;
#7521=CARTESIAN_POINT ( 'NONE',  ( -13.14518615778179544, 34.20351562608393436, 0.000000000000000000 ) ) ;
#7522=CARTESIAN_POINT ( 'NONE',  ( 13.57481594606304931, 35.89023437716787868, 5.622872871577869525 ) ) ;
#7535=CARTESIAN_POINT ( 'NONE',  ( 0.000000000000000000, 1.000000000000000000, 0.000000000000000000 ) ) ;
#7548=CARTESIAN_POINT ( 'NONE',  ( -9.295050272127044266, 36.08867187608393579, 9.295050272127047819 ) ) ;
#7573=VECTOR ( 'NONE', #22992, 1000.000000000000000 ) ;
#7580=CARTESIAN_POINT ( 'NONE',  ( -9.295050272127046043, 37.27929687608393294, -9.295050272127046043 ) ) ;
#7622=EDGE_CURVE ( 'NONE', #25304, #12136, #16717, .T. ) ;
#7630=CARTESIAN_POINT ( 'NONE',  ( 0.000000000000000000, -1.000000000000001998, 0.000000000000000000 ) ) ;
#7652=CARTESIAN_POINT ( 'NONE',  ( 0.000000000000000000, 10.00000000000000000, 19.22649730810373470 ) ) ;
#7664=CARTESIAN_POINT ( 'NONE',  ( -8.312177448680279460E-16, 35.24531249999999716, -13.57481594606304576 ) ) ;
#7666=CARTESIAN_POINT ( 'NONE',  ( 13.57481594606304576, 39.80937499999999574, -1.662435489736055892E-15 ) ) ;
#7669=CARTESIAN_POINT ( 'NONE',  ( 5.622872871577878406, 37.37851562716787157, 13.57481594606304576 ) ) ;
#7693=CARTESIAN_POINT ( 'NONE',  ( 5.444914386472302859, 33.06250000108393294, 13.14518615778179189 ) ) ;
#7724=CARTESIAN_POINT ( 'NONE',  ( 13.14518615778179900, 33.85625000108393579, -5.444914386472297529 ) ) ;
#7733=ORIENTED_EDGE ( 'NONE', *, *, #22456, .F. ) ;
#7770=CARTESIAN_POINT ( 'NONE',  ( -5.622872871577920151, 35.69179687716787441, 13.57481594606300135 ) ) ;
#7774=CARTESIAN_POINT ( 'NONE',  ( 0.000000000000000000, 36.00000000000000000, 0.000000000000000000 ) ) ;
#7775=CARTESIAN_POINT ( 'NONE',  ( -5.444914386472297529, 39.80937500108392868, -13.14518615778179900 ) ) ;
#7798=DIRECTION ( 'NONE',  ( -0.000000000000000000, -1.000000000000000000, -0.000000000000000000 ) ) ;
#7807=CARTESIAN_POINT ( 'NONE',  ( -6.470563696665745823, 36.00000000000002132, -11.78199955157067080 ) ) ;
#7808=CARTESIAN_POINT ( 'NONE',  ( -5.622872871577873077, 40.05742187499999574, -13.57481594606304753 ) ) ;
#7810=CARTESIAN_POINT ( 'NONE',  ( 13.14518615778179544, 32.21914062608393436, -1.609821015232357215E-15 ) ) ;
#7811=CARTESIAN_POINT ( 'NONE',  ( -13.57481594606304576, 33.95546875216787441, 0.000000000000000000 ) ) ;
#7832=CARTESIAN_POINT ( 'NONE',  ( 9.295050272127047819, 33.11210937608393579, 9.295050272127046043 ) ) ;
#7856=( BOUNDED_CURVE ( )  B_SPLINE_CURVE ( 2, ( #1123, #20206, #5106, #11776, #4970, #16058, #26776, #16205, #24909 ),
 .UNSPECIFIED., .F., .F. ) 
 B_SPLINE_CURVE_WITH_KNOTS ( ( 3, 2, 2, 2, 3 ),
 ( 0.7291666666666668517, 0.7395833333333334814, 0.7500000000000001110, 0.7604166666666667407, 0.7708333333333333703 ),
 .UNSPECIFIED. ) 
 CURVE ( )  GEOMETRIC_REPRESENTATION_ITEM ( )  RATIONAL_B_SPLINE_CURVE ( ( 0.9999999999999983347, 0.9238795325112884038, 1.000000000000000000, 0.9238795325112867385, 1.000000000000000000, 0.9238795325112867385, 1.000000000000000000, 0.9238795325112867385, 1.000000000000000000 ) ) 
 REPRESENTATION_ITEM ( '' )  );
#7864=CARTESIAN_POINT ( 'NONE',  ( -5.444914386472299306, 32.76484375108393010, 13.14518615778179722 ) ) ;
#7871=CONICAL_SURFACE ( 'NONE', #8330, 23.85284712729792389, 0.9599310885968833640 ) ;
#7876=CARTESIAN_POINT ( 'NONE',  ( 5.444914386472297529, 35.54296875108393294, -13.14518615778179900 ) ) ;
#7902=ORIENTED_EDGE ( 'NONE', *, *, #20337, .F. ) ;
#7911=CARTESIAN_POINT ( 'NONE',  ( -5.444914386472297529, 40.60312500108393863, -13.14518615778179900 ) ) ;
#7925=ADVANCED_FACE ( 'NONE', ( #27119 ), #1811, .F. ) ;
#7933=ADVANCED_FACE ( 'NONE', ( #5448 ), #22298, .T. ) ;
#7942=CARTESIAN_POINT ( 'NONE',  ( -13.57481594606304576, 40.99999999999999289, 0.000000000000000000 ) ) ;
#7945=CARTESIAN_POINT ( 'NONE',  ( -9.598844408820458085, 31.47500000216787441, -9.598844408820458085 ) ) ;
#7962=ORIENTED_EDGE ( 'NONE', *, *, #4299, .T. ) ;
#7965=CARTESIAN_POINT ( 'NONE',  ( -13.14518615778179189, 32.86406250108393579, 5.444914386472304635 ) ) ;
#7988=VECTOR ( 'NONE', #2194, 1000.000000000000000 ) ;
#7997=CARTESIAN_POINT ( 'NONE',  ( 9.295050272127047819, 32.91367187608393152, 9.295050272127046043 ) ) ;
#8003=ORIENTED_EDGE ( 'NONE', *, *, #4147, .T. ) ;
#8012=CARTESIAN_POINT ( 'NONE',  ( 5.444914386472302859, 32.86406250108392868, 13.14518615778179189 ) ) ;
#8035=AXIS2_PLACEMENT_3D ( 'NONE', #26816, #13951, #7404 ) ;
#8041=CIRCLE ( 'NONE', #20348, 25.00000000000000711 ) ;
#8043=CARTESIAN_POINT ( 'NONE',  ( 5.622872871577786924, 33.40976562716787157, 13.57481594606313813 ) ) ;
#8075=CARTESIAN_POINT ( 'NONE',  ( -9.598844408820458085, 32.16953124999999147, -9.598844408820458085 ) ) ;
#8079=CARTESIAN_POINT ( 'NONE',  ( 5.622872871577871301, 39.16445312499999432, -13.57481594606304753 ) ) ;
#8081=CARTESIAN_POINT ( 'NONE',  ( 5.622872871577871301, 33.70742187716787441, -13.57481594606304753 ) ) ;
#8102=ORIENTED_EDGE ( 'NONE', *, *, #16815, .F. ) ;
#8106=CARTESIAN_POINT ( 'NONE',  ( -8.049105076161786076E-16, 31.82226562608393650, -13.14518615778179544 ) ) ;
#8108=CARTESIAN_POINT ( 'NONE',  ( 2.493653234604083739E-15, 34.94765625216787441, 13.57481594606304576 ) ) ;
#8124=CARTESIAN_POINT ( 'NONE',  ( -1.021803718759008106, 36.00000000000000000, 13.11239906893445806 ) ) ;
#8140=CARTESIAN_POINT ( 'NONE',  ( -5.444914386472299306, 33.55859375108393294, 13.14518615778179722 ) ) ;
#8156=CARTESIAN_POINT ( 'NONE',  ( 2.414731522848535132E-15, 32.02070312608393010, 13.14518615778179544 ) ) ;
#8164=CARTESIAN_POINT ( 'NONE',  ( 13.57481594606304931, 31.92148437716787157, 5.622872871577868636 ) ) ;
#8167=MECHANICAL_DESIGN_GEOMETRIC_PRESENTATION_REPRESENTATION('',(#20468),#15881);
#8182=( BOUNDED_CURVE ( )  B_SPLINE_CURVE ( 1, ( #13776, #2963 ),
 .UNSPECIFIED., .F., .F. ) 
 B_SPLINE_CURVE_WITH_KNOTS ( ( 2, 2 ),
 ( 0.000000000000000000, 1.000000000000000000 ),
 .UNSPECIFIED. ) 
 CURVE ( )  GEOMETRIC_REPRESENTATION_ITEM ( )  RATIONAL_B_SPLINE_CURVE ( ( 0.9684275710300105366, 0.9684275710300105366 ) ) 
 REPRESENTATION_ITEM ( '' )  );
#8187=CARTESIAN_POINT ( 'NONE',  ( 13.57481594606304753, 34.40195312716787157, -5.622872871577873966 ) ) ;
#8212=SURFACE_STYLE_FILL_AREA ( #14750 ) ;
#8216=CARTESIAN_POINT ( 'NONE',  ( 13.14518615778179544, 32.41757812608393863, -1.609821015232357215E-15 ) ) ;
#8217=CARTESIAN_POINT ( 'NONE',  ( 13.14518615778179722, 32.16953125108393152, 5.444914386472293977 ) ) ;
#8218=CARTESIAN_POINT ( 'NONE',  ( 5.622872871577871301, 34.50117187716788436, -13.57481594606304753 ) ) ;
#8242=CARTESIAN_POINT ( 'NONE',  ( 12.07727640983550188, 36.00000000000000711, -6.197985357349471869 ) ) ;
#8244=CARTESIAN_POINT ( 'NONE',  ( 7.279598927625384519, 35.96878166309014802, -11.91808989001553520 ) ) ;
#8271=VERTEX_POINT ( 'NONE', #14633 ) ;
#8272=CARTESIAN_POINT ( 'NONE',  ( 5.444914386472302859, 32.86406250108392868, 13.14518615778179189 ) ) ;
#8289=CARTESIAN_POINT ( 'NONE',  ( 13.14518615778179900, 33.75703125108393010, 5.444914386472293977 ) ) ;
#8312=CARTESIAN_POINT ( 'NONE',  ( -8.312177448680279460E-16, 34.55078125216787299, -13.57481594606304576 ) ) ;
#8330=AXIS2_PLACEMENT_3D ( 'NONE', #14308, #21163, #14450 ) ;
#8354=FACE_OUTER_BOUND ( 'NONE', #27508, .T. ) ;
#8356=CARTESIAN_POINT ( 'NONE',  ( 9.295050272127047819, 32.11992187608393579, 9.295050272127046043 ) ) ;
#8357=CARTESIAN_POINT ( 'NONE',  ( 9.598844408820456309, 32.07031250216787299, -9.598844408820458085 ) ) ;
#8386=LINE ( 'NONE', #2125, #15702 ) ;
#8395=CARTESIAN_POINT ( 'NONE',  ( -12.05655202970020312, 36.00000000000000000, 5.307619621752285965 ) ) ;
#8400=AXIS2_PLACEMENT_3D ( 'NONE', #10023, #21016, #6043 ) ;
#8409=CARTESIAN_POINT ( 'NONE',  ( -13.14518615778179722, 35.14609375108393152, -5.444914386472297529 ) ) ;
#8410=CARTESIAN_POINT ( 'NONE',  ( 6.944426393311538881, 31.55306875057403104, -11.16113171639042356 ) ) ;
#8423=( BOUNDED_CURVE ( )  B_SPLINE_CURVE ( 2, ( #21531, #19383, #10255, #8, #19107, #4146, #14670, #21254, #18965 ),
 .UNSPECIFIED., .F., .T. ) 
 B_SPLINE_CURVE_WITH_KNOTS ( ( 3, 2, 2, 2, 3 ),
 ( 0.8541666666666662966, 0.8645833333333331483, 0.8750000000000000000, 0.8854166666666667407, 0.8958333333333335924 ),
 .UNSPECIFIED. ) 
 CURVE ( )  GEOMETRIC_REPRESENTATION_ITEM ( )  RATIONAL_B_SPLINE_CURVE ( ( 1.000000000000002442, 0.9238795325112842960, 1.000000000000000000, 0.9238795325112867385, 1.000000000000000000, 0.9238795325112867385, 1.000000000000000000, 0.9238795325112850731, 1.000000000000001554 ) ) 
 REPRESENTATION_ITEM ( '' )  );
#8428=DIRECTION ( 'NONE',  ( 0.000000000000000000, 0.000000000000000000, 1.000000000000000000 ) ) ;
#8436=CARTESIAN_POINT ( 'NONE',  ( 13.57481594606304753, 35.09648437499999574, -5.622872871577873966 ) ) ;
#8455=CARTESIAN_POINT ( 'NONE',  ( -5.622872871577737186, 34.89804687716787157, 13.57481594606318254 ) ) ;
#8501=CARTESIAN_POINT ( 'NONE',  ( -8.049105076161786076E-16, 40.35507812608393152, -13.14518615778179544 ) ) ;
#8531=CARTESIAN_POINT ( 'NONE',  ( -13.14518615778179900, 38.32109375108394289, -5.444914386472297529 ) ) ;
#8543=ORIENTED_EDGE ( 'NONE', *, *, #18490, .F. ) ;
#8554=CARTESIAN_POINT ( 'NONE',  ( -5.444914386472299306, 34.55078125108393294, 13.14518615778179722 ) ) ;
#8555=CARTESIAN_POINT ( 'NONE',  ( -8.049105076161786076E-16, 39.75976562608394005, -13.14518615778179544 ) ) ;
#8593=CARTESIAN_POINT ( 'NONE',  ( -5.622872871577965448, 34.00507812499998295, 13.57481594606295161 ) ) ;
#8596=EDGE_CURVE ( 'NONE', #18417, #8271, #7265, .T. ) ;
#8597=CARTESIAN_POINT ( 'NONE',  ( -13.57481594606304753, 34.69960937716787441, -5.622872871577872189 ) ) ;
#8614=VERTEX_POINT ( 'NONE', #24614 ) ;
#8626=CARTESIAN_POINT ( 'NONE',  ( 13.14518615778179544, 33.21132812608393436, -1.609821015232357215E-15 ) ) ;
#8632=AXIS2_PLACEMENT_3D ( 'NONE', #16262, #17979, #27258 ) ;
#8635=CARTESIAN_POINT ( 'NONE',  ( 0.000000000000000000, 0.000000000000000000, 0.000000000000000000 ) ) ;
#8637=VERTEX_POINT ( 'NONE', #9216 ) ;
#8643=CARTESIAN_POINT ( 'NONE',  ( 3.878385410779738418, 31.34156310770110565, -13.57481594606304931 ) ) ;
#8649=ORIENTED_EDGE ( 'NONE', *, *, #13672, .F. ) ;
#8658=CARTESIAN_POINT ( 'NONE',  ( 12.25119088044477600, 35.99999999999998579, 5.405483146087242119 ) ) ;
#8667=CARTESIAN_POINT ( 'NONE',  ( 0.000000000000000000, 10.00000000000000178, 0.000000000000000000 ) ) ;
#8669=CARTESIAN_POINT ( 'NONE',  ( 13.57481594606304931, 35.79101562499999289, 5.622872871577869525 ) ) ;
#8671=CARTESIAN_POINT ( 'NONE',  ( -13.14518615778179544, 35.98945312608393721, 0.000000000000000000 ) ) ;
#8696=CARTESIAN_POINT ( 'NONE',  ( 5.444914386472297529, 34.15390625108393863, -13.14518615778179722 ) ) ;
#8697=CARTESIAN_POINT ( 'NONE',  ( -13.14518615778179900, 39.11484375108394573, -5.444914386472297529 ) ) ;
#8737=ORIENTED_EDGE ( 'NONE', *, *, #22715, .F. ) ;
#8758=AXIS2_PLACEMENT_3D ( 'NONE', #5983, #3985, #25369 ) ;
#8760=EDGE_CURVE ( 'NONE', #13376, #21990, #9268, .T. ) ;
#8761=( BOUNDED_CURVE ( )  B_SPLINE_CURVE ( 1, ( #26035, #28043 ),
 .UNSPECIFIED., .F., .F. ) 
 B_SPLINE_CURVE_WITH_KNOTS ( ( 2, 2 ),
 ( 0.000000000000000000, 1.000000000000000000 ),
 .UNSPECIFIED. ) 
 CURVE ( )  GEOMETRIC_REPRESENTATION_ITEM ( )  RATIONAL_B_SPLINE_CURVE ( ( 0.9684275895297407288, 0.9684275895297407288 ) ) 
 REPRESENTATION_ITEM ( '' )  );
#8778=CARTESIAN_POINT ( 'NONE',  ( -9.295050272127046043, 38.07304687608393579, -9.295050272127046043 ) ) ;
#8809=CARTESIAN_POINT ( 'NONE',  ( 2.493653234604083739E-15, 37.22968749999999716, 13.57481594606304576 ) ) ;
#8811=CARTESIAN_POINT ( 'NONE',  ( 13.14518615778179544, 36.38632812608393863, -1.609821015232357215E-15 ) ) ;
#8838=CARTESIAN_POINT ( 'NONE',  ( 5.444914386472297529, 35.74140625108393721, -13.14518615778179722 ) ) ;
#8839=CARTESIAN_POINT ( 'NONE',  ( -5.444914386472299306, 38.51953125108393294, 13.14518615778179722 ) ) ;
#8851=AXIS2_PLACEMENT_3D ( 'NONE', #16118, #11836, #24687 ) ;
#8854=FACE_OUTER_BOUND ( 'NONE', #11940, .T. ) ;
#8864=VERTEX_POINT ( 'NONE', #5517 ) ;
#8920=CARTESIAN_POINT ( 'NONE',  ( -13.14518615778179189, 39.80937500108392868, 5.444914386472304635 ) ) ;
#8937=CARTESIAN_POINT ( 'NONE',  ( 6.831134457305117813, 36.00000000000001421, 11.35217666745981369 ) ) ;
#8950=CARTESIAN_POINT ( 'NONE',  ( 13.57481594606304753, 38.27148437500000711, -5.622872871577873077 ) ) ;
#8953=CARTESIAN_POINT ( 'NONE',  ( -13.14518615778179544, 37.57695312608393579, 0.000000000000000000 ) ) ;
#8977=CARTESIAN_POINT ( 'NONE',  ( 2.493653234604083739E-15, 32.56640625216787299, 13.57481594606304576 ) ) ;
#8981=CARTESIAN_POINT ( 'NONE',  ( 13.14518615778179544, 39.56132812608393579, -1.609821015232357215E-15 ) ) ;
#8999=CARTESIAN_POINT ( 'NONE',  ( 2.493653234604083739E-15, 34.84843749999999574, 13.57481594606304576 ) ) ;
#9009=DIRECTION ( 'NONE',  ( -0.000000000000000000, -1.000000000000000000, -0.000000000000000000 ) ) ;
#9017=CARTESIAN_POINT ( 'NONE',  ( -9.295050272127046043, 39.66054687608393436, -9.295050272127046043 ) ) ;
#9064=CARTESIAN_POINT ( 'NONE',  ( -13.14518615778179544, 36.58476562608393579, 0.000000000000000000 ) ) ;
#9085=DIRECTION ( 'NONE',  ( 0.000000000000000000, 0.000000000000000000, 1.000000000000000000 ) ) ;
#9091=ORIENTED_EDGE ( 'NONE', *, *, #14686, .T. ) ;
#9093=CARTESIAN_POINT ( 'NONE',  ( 0.000000000000000000, 23.00000000000000000, 0.000000000000000000 ) ) ;
#9095=CARTESIAN_POINT ( 'NONE',  ( 2.493653234604083739E-15, 38.02343749999999289, 13.57481594606304576 ) ) ;
#9097=CARTESIAN_POINT ( 'NONE',  ( 5.444914386472302859, 36.23750000108393721, 13.14518615778179189 ) ) ;
#9123=CARTESIAN_POINT ( 'NONE',  ( 13.14518615778179900, 35.64218750108393152, -5.444914386472297529 ) ) ;
#9145=SHAPE_REPRESENTATION ( 'Suction Cups Set (x4)', ( #26844 ), #17253 ) ;
#9151=EDGE_CURVE ( 'NONE', #10542, #20304, #13923, .T. ) ;
#9157=FACE_OUTER_BOUND ( 'NONE', #5559, .T. ) ;
#9168=DIRECTION ( 'NONE',  ( -1.000000000000000000, 0.000000000000000000, 0.000000000000000000 ) ) ;
#9169=ORIENTED_EDGE ( 'NONE', *, *, #14543, .F. ) ;
#9173=CARTESIAN_POINT ( 'NONE',  ( 0.000000000000000000, 20.53589838486225361, 23.00000000000001421 ) ) ;
#9187=EDGE_LOOP ( 'NONE', ( #23937, #19249, #19062, #17736, #14281, #3652, #19700, #18386, #12753, #26619, #660, #5918, #6357, #27951, #8737, #4285 ) ) ;
#9202=DIRECTION ( 'NONE',  ( -0.000000000000000000, -1.000000000000000000, -0.000000000000000000 ) ) ;
#9203=CARTESIAN_POINT ( 'NONE',  ( 9.295050272127047819, 35.29492187608393294, 9.295050272127046043 ) ) ;
#9216=CARTESIAN_POINT ( 'NONE',  ( -8.312177448680279460E-16, 34.55078125216787299, -13.57481594606304576 ) ) ;
#9225=CARTESIAN_POINT ( 'NONE',  ( 0.000000000000000000, 36.00000000000000000, 0.000000000000000000 ) ) ;
#9227=CARTESIAN_POINT ( 'NONE',  ( 13.57481594606304753, 39.95820312716787726, -5.622872871577873077 ) ) ;
#9236=CARTESIAN_POINT ( 'NONE',  ( 5.622872871577871301, 35.98945312499999716, -13.57481594606304753 ) ) ;
#9238=CARTESIAN_POINT ( 'NONE',  ( 2.414731522848535132E-15, 34.60039062608393579, 13.14518615778179544 ) ) ;
#9241=CARTESIAN_POINT ( 'NONE',  ( 13.57481594606304931, 37.47773437716787726, 5.622872871577869525 ) ) ;
#9262=CARTESIAN_POINT ( 'NONE',  ( -13.14518615778179900, 35.14609375108393152, -5.444914386472297529 ) ) ;
#9268=( BOUNDED_CURVE ( )  B_SPLINE_CURVE ( 2, ( #5654, #17128, #23040 ),
 .UNSPECIFIED., .F., .F. ) 
 B_SPLINE_CURVE_WITH_KNOTS ( ( 3, 3 ),
 ( 0.9375000000000000000, 0.9448586968893691873 ),
 .UNSPECIFIED. ) 
 CURVE ( )  GEOMETRIC_REPRESENTATION_ITEM ( )  RATIONAL_B_SPLINE_CURVE ( ( 1.000000000000000000, 0.9462258450566536361, 0.9684275698016389100 ) ) 
 REPRESENTATION_ITEM ( '' )  );
#9291=CARTESIAN_POINT ( 'NONE',  ( -9.295050272127044266, 36.68398437608392726, 9.295050272127047819 ) ) ;
#9330=CARTESIAN_POINT ( 'NONE',  ( -13.57481594606304753, 33.90585937716787868, -5.622872871577872189 ) ) ;
#9340=CARTESIAN_POINT ( 'NONE',  ( 5.444914386472297529, 34.74921875108394431, -13.14518615778179900 ) ) ;
#9364=CARTESIAN_POINT ( 'NONE',  ( -13.57481594606304753, 40.25585937716787299, -5.622872871577873077 ) ) ;
#9369=CARTESIAN_POINT ( 'NONE',  ( -13.57481594606304398, 35.49335937499999005, 5.622872871577880183 ) ) ;
#9371=CARTESIAN_POINT ( 'NONE',  ( -5.622872871577873077, 33.70742187500000142, -13.57481594606304753 ) ) ;
#9373=CARTESIAN_POINT ( 'NONE',  ( 13.14518615778179544, 33.21132812608393436, -1.609821015232357215E-15 ) ) ;
#9375=CARTESIAN_POINT ( 'NONE',  ( 13.14518615778179722, 34.65000000108393152, -5.444914386472297529 ) ) ;
#9376=CARTESIAN_POINT ( 'NONE',  ( -9.598844408820454532, 34.84843750216787583, 9.598844408820459861 ) ) ;
#9382=( BOUNDED_SURFACE ( )  B_SPLINE_SURFACE ( 1, 2, ( 
 ( #26752, #20753, #14177, #7911, #27449, #25157, #5648, #9901, #12308, #3359, #12030, #27319, #16605, #14453, #16463, #18613, #1238, #25298, #23170, #7775, #12165, #14310, #23032, #20893, #3504, #1376, #16328, #10037, #18749, #5786, #5510, #25027, #3645, #22895, #6665, #26350, #2127, #26494, #23649, #13058, #19643, #12920, #15066, #6809, #22077, #26059, #4688, #21795, #15350, #8531, #1988, #17501, #15205, #19786, #26201, #268, #23925, #17792, #4124, #15497, #25922, #24209, #2274, #10933, #8953, #24066, #13348, #12789, #21938, #17643, #10654, #2554, #11214, #21507, #4542, #19930, #13204, #14929, #2415, #6527, #28065, #19362, #17217, #4404, #413, #126, #11074, #6396, #8811, #10792, #23783, #9097, #4259, #21652, #19506, #20429, #8671, #17363, #13919, #11639, #26784, #15787, #7229, #7519, #990, #4975, #11355, #18069, #847, #5112, #11784, #15920, #20507, #24636, #13640, #16066, #13777, #11925, #2964, #11498, #22788, #24490, #27068, #9799, #9238, #24915, #9658, #16214, #18505, #22355, #18219, #5399, #15646, #18360, #14068, #2830, #22499, #20362, #9520, #20215, #6951, #24344, #20647, #3258, #1130, #700, #26928, #7371, #556, #4835, #13496, #22647, #9373, #22216, #24774, #2694, #20078, #17930, #26640, #7087, #5255, #3116, #12472, #20785, #16639, #14487, #3389, #1681, #8216, #1266, #14620, #21198, #9930, #19048, #23337, #27486, #10340, #27756, #16906, #25603, #3540, #21340, #27621 ),
 ( #7942, #23204, #14755, #6088, #25474, #23475, #3812, #10067, #3954, #21060, #25193, #12060, #25331, #18645, #5817, #5544, #18779, #1818, #14208, #7808, #12613, #27211, #27350, #10484, #7666, #12343, #16358, #16498, #25058, #22928, #3679, #5680, #14347, #23062, #12197, #20925, #1408, #8079, #1549, #10201, #18911, #16774, #5953, #6663, #11073, #11353, #15644, #26492, #266, #26638, #12918, #13493, #26348, #15203, #19641, #8950, #13346, #28202, #4401, #10790, #9095, #411, #4540, #13202, #2272, #15065, #26057, #6525, #17499, #6949, #2692, #15348, #124, #21792, #24342, #554, #8809, #6807, #23923, #19783, #15495, #13056, #24206, #17928, #4686, #26198, #21936, #21650, #23780, #10931, #4833, #22075, #22213, #24063, #4257, #2124, #2413, #17641, #2552, #11211, #20075, #9236, #19928, #19504, #17789, #8669, #17361, #22353, #9656, #7369, #11923, #18358, #20645, #16064, #9927, #15783, #7664, #18066, #18504, #13918, #3114, #1128, #7517, #27210, #24488, #14066, #9797, #2828, #5541, #16356, #13638, #27066, #25055, #16211, #18642, #24914, #18216, #20212, #11496, #698, #24772, #14204, #26926, #5397, #26782, #7085, #845, #9371, #7227, #5253, #11782, #22925, #22645, #24634, #3386, #12056, #15918, #22786, #20782, #3256, #4973, #1264, #20505, #5110, #13775, #22497, #988, #2962, #11637, #20359, #9518, #27347, #21058, #12193, #5677, #10197, #23334, #25741, #8075, #16635, #25471, #1679, #27483 ) ),
 .UNSPECIFIED., .F., .F., .T. ) 
 B_SPLINE_SURFACE_WITH_KNOTS ( ( 2, 2 ),
 ( 3, 2, 2, 2, 2, 2, 2, 2, 2, 2, 2, 2, 2, 2, 2, 2, 2, 2, 2, 2, 2, 2, 2, 2, 2, 2, 2, 2, 2, 2, 2, 2, 2, 2, 2, 2, 2, 2, 2, 2, 2, 2, 2, 2, 2, 2, 2, 2, 2, 2, 2, 2, 2, 2, 2, 2, 2, 2, 2, 2, 2, 2, 2, 2, 2, 2, 2, 2, 2, 2, 2, 2, 2, 2, 2, 2, 2, 2, 2, 2, 2, 2, 2, 2, 2, 2, 2, 2, 2, 2, 2, 3 ),
 ( 0.000000000000000000, 1.000000000000000000 ),
 ( 0.000000000000000000, 0.01041666666666666609, 0.02083333333333333218, 0.03125000000000000000, 0.04166666666666666435, 0.05208333333333333565, 0.06250000000000000000, 0.07291666666666667129, 0.08333333333333332871, 0.09375000000000000000, 0.1041666666666666713, 0.1145833333333333287, 0.1250000000000000000, 0.1354166666666666574, 0.1458333333333333426, 0.1562500000000000000, 0.1666666666666666574, 0.1770833333333333426, 0.1875000000000000000, 0.1979166666666666574, 0.2083333333333333426, 0.2187500000000000000, 0.2291666666666666574, 0.2395833333333333426, 0.2500000000000000000, 0.2604166666666666852, 0.2708333333333333148, 0.2812500000000000000, 0.2916666666666666852, 0.3020833333333333148, 0.3125000000000000000, 0.3229166666666666852, 0.3333333333333333148, 0.3437500000000000000, 0.3541666666666666852, 0.3645833333333333148, 0.3750000000000000000, 0.3854166666666666852, 0.3958333333333333148, 0.4062500000000000000, 0.4166666666666666852, 0.4270833333333333148, 0.4375000000000000000, 0.4479166666666666852, 0.4583333333333333148, 0.4687500000000000000, 0.4791666666666666852, 0.4895833333333333148, 0.5000000000000000000, 0.5104166666666666297, 0.5208333333333333703, 0.5312500000000000000, 0.5416666666666666297, 0.5520833333333333703, 0.5625000000000000000, 0.5729166666666666297, 0.5833333333333333703, 0.5937500000000000000, 0.6041666666666666297, 0.6145833333333333703, 0.6250000000000000000, 0.6354166666666666297, 0.6458333333333333703, 0.6562500000000000000, 0.6666666666666666297, 0.6770833333333333703, 0.6875000000000000000, 0.6979166666666666297, 0.7083333333333333703, 0.7187500000000000000, 0.7291666666666666297, 0.7395833333333333703, 0.7500000000000000000, 0.7604166666666666297, 0.7708333333333333703, 0.7812500000000000000, 0.7916666666666666297, 0.8020833333333333703, 0.8125000000000000000, 0.8229166666666666297, 0.8333333333333333703, 0.8437500000000000000, 0.8541666666666666297, 0.8645833333333333703, 0.8750000000000000000, 0.8854166666666666297, 0.8958333333333333703, 0.9062500000000000000, 0.9166666666666666297, 0.9270833333333333703, 0.9375000000000000000, 0.9448586968893691873 ),
 .UNSPECIFIED. ) 
 GEOMETRIC_REPRESENTATION_ITEM ( )  RATIONAL_B_SPLINE_SURFACE ( (
 ( 1.000000000000000000, 0.9238795325112867385, 1.000000000000000000, 0.9238795325112867385, 1.000000000000000000, 0.9238795325112867385, 1.000000000000000000, 0.9238795325112867385, 1.000000000000000000, 0.9238795325112867385, 1.000000000000000000, 0.9238795325112867385, 1.000000000000000000, 0.9238795325112867385, 1.000000000000000000, 0.9238795325112867385, 1.000000000000000000, 0.9238795325112867385, 1.000000000000000000, 0.9238795325112867385, 1.000000000000000000, 0.9238795325112867385, 1.000000000000000000, 0.9238795325112867385, 1.000000000000000000, 0.9238795325112867385, 1.000000000000000000, 0.9238795325112867385, 1.000000000000000000, 0.9238795325112867385, 1.000000000000000000, 0.9238795325112867385, 1.000000000000000000, 0.9238795325112867385, 1.000000000000000000, 0.9238795325112867385, 1.000000000000000000, 0.9238795325112867385, 1.000000000000000000, 0.9238795325112867385, 1.000000000000000000, 0.9238795325112867385, 1.000000000000000000, 0.9238795325112867385, 1.000000000000000000, 0.9238795325112867385, 1.000000000000000000, 0.9238795325112867385, 1.000000000000000000, 0.9238795325112867385, 1.000000000000000000, 0.9238795325112867385, 1.000000000000000000, 0.9238795325112867385, 1.000000000000000000, 0.9238795325112867385, 1.000000000000000000, 0.9238795325112867385, 1.000000000000000000, 0.9238795325112867385, 1.000000000000000000, 0.9238795325112867385, 1.000000000000000000, 0.9238795325112867385, 1.000000000000000000, 0.9238795325112867385, 1.000000000000000000, 0.9238795325112867385, 1.000000000000000000, 0.9238795325112867385, 1.000000000000000000, 0.9238795325112867385, 1.000000000000000000, 0.9238795325112867385, 1.000000000000000000, 0.9238795325112867385, 1.000000000000000000, 0.9238795325112867385, 1.000000000000000000, 0.9238795325112867385, 1.000000000000000000, 0.9238795325112867385, 1.000000000000000000, 0.9238795325112867385, 1.000000000000000000, 0.9238795325112867385, 1.000000000000000000, 0.9238795325112867385, 1.000000000000000000, 0.9238795325112867385, 1.000000000000000000, 0.9238795325112867385, 1.000000000000000000, 0.9238795325112867385, 1.000000000000000000, 0.9238795325112867385, 1.000000000000000000, 0.9238795325112867385, 1.000000000000000000, 0.9238795325112867385, 1.000000000000000000, 0.9238795325112867385, 1.000000000000000000, 0.9238795325112867385, 1.000000000000000000, 0.9238795325112867385, 1.000000000000000000, 0.9238795325112867385, 1.000000000000000000, 0.9238795325112867385, 1.000000000000000000, 0.9238795325112867385, 1.000000000000000000, 0.9238795325112867385, 1.000000000000000000, 0.9238795325112867385, 1.000000000000000000, 0.9238795325112867385, 1.000000000000000000, 0.9238795325112867385, 1.000000000000000000, 0.9238795325112867385, 1.000000000000000000, 0.9238795325112867385, 1.000000000000000000, 0.9238795325112867385, 1.000000000000000000, 0.9238795325112867385, 1.000000000000000000, 0.9238795325112867385, 1.000000000000000000, 0.9238795325112867385, 1.000000000000000000, 0.9238795325112867385, 1.000000000000000000, 0.9238795325112867385, 1.000000000000000000, 0.9238795325112867385, 1.000000000000000000, 0.9238795325112867385, 1.000000000000000000, 0.9238795325112867385, 1.000000000000000000, 0.9238795325112867385, 1.000000000000000000, 0.9238795325112867385, 1.000000000000000000, 0.9238795325112867385, 1.000000000000000000, 0.9238795325112867385, 1.000000000000000000, 0.9238795325112867385, 1.000000000000000000, 0.9238795325112867385, 1.000000000000000000, 0.9238795325112867385, 1.000000000000000000, 0.9238795325112867385, 1.000000000000000000, 0.9238795325112867385, 1.000000000000000000, 0.9238795325112867385, 1.000000000000000000, 0.9238795325112867385, 1.000000000000000000, 0.9238795325112867385, 1.000000000000000000, 0.9238795325112867385, 1.000000000000000000, 0.9238795325112867385, 1.000000000000000000, 0.9238795325112867385, 1.000000000000000000, 0.9238795325112867385, 1.000000000000000000, 0.9238795325112867385, 1.000000000000000000, 0.9238795325112867385, 1.000000000000000000, 0.9238795325112867385, 1.000000000000000000, 0.9462258450566536361, 0.9684275698016389100),
 ( 1.000000000000000000, 0.9238795325112867385, 1.000000000000000000, 0.9238795325112867385, 1.000000000000000000, 0.9238795325112867385, 1.000000000000000000, 0.9238795325112867385, 1.000000000000000000, 0.9238795325112867385, 1.000000000000000000, 0.9238795325112867385, 1.000000000000000000, 0.9238795325112867385, 1.000000000000000000, 0.9238795325112867385, 1.000000000000000000, 0.9238795325112867385, 1.000000000000000000, 0.9238795325112867385, 1.000000000000000000, 0.9238795325112867385, 1.000000000000000000, 0.9238795325112867385, 1.000000000000000000, 0.9238795325112867385, 1.000000000000000000, 0.9238795325112867385, 1.000000000000000000, 0.9238795325112867385, 1.000000000000000000, 0.9238795325112867385, 1.000000000000000000, 0.9238795325112867385, 1.000000000000000000, 0.9238795325112867385, 1.000000000000000000, 0.9238795325112867385, 1.000000000000000000, 0.9238795325112867385, 1.000000000000000000, 0.9238795325112867385, 1.000000000000000000, 0.9238795325112867385, 1.000000000000000000, 0.9238795325112867385, 1.000000000000000000, 0.9238795325112867385, 1.000000000000000000, 0.9238795325112867385, 1.000000000000000000, 0.9238795325112867385, 1.000000000000000000, 0.9238795325112867385, 1.000000000000000000, 0.9238795325112867385, 1.000000000000000000, 0.9238795325112867385, 1.000000000000000000, 0.9238795325112867385, 1.000000000000000000, 0.9238795325112867385, 1.000000000000000000, 0.9238795325112867385, 1.000000000000000000, 0.9238795325112867385, 1.000000000000000000, 0.9238795325112867385, 1.000000000000000000, 0.9238795325112867385, 1.000000000000000000, 0.9238795325112867385, 1.000000000000000000, 0.9238795325112867385, 1.000000000000000000, 0.9238795325112867385, 1.000000000000000000, 0.9238795325112867385, 1.000000000000000000, 0.9238795325112867385, 1.000000000000000000, 0.9238795325112867385, 1.000000000000000000, 0.9238795325112867385, 1.000000000000000000, 0.9238795325112867385, 1.000000000000000000, 0.9238795325112867385, 1.000000000000000000, 0.9238795325112867385, 1.000000000000000000, 0.9238795325112867385, 1.000000000000000000, 0.9238795325112867385, 1.000000000000000000, 0.9238795325112867385, 1.000000000000000000, 0.9238795325112867385, 1.000000000000000000, 0.9238795325112867385, 1.000000000000000000, 0.9238795325112867385, 1.000000000000000000, 0.9238795325112867385, 1.000000000000000000, 0.9238795325112867385, 1.000000000000000000, 0.9238795325112867385, 1.000000000000000000, 0.9238795325112867385, 1.000000000000000000, 0.9238795325112867385, 1.000000000000000000, 0.9238795325112867385, 1.000000000000000000, 0.9238795325112867385, 1.000000000000000000, 0.9238795325112867385, 1.000000000000000000, 0.9238795325112867385, 1.000000000000000000, 0.9238795325112867385, 1.000000000000000000, 0.9238795325112867385, 1.000000000000000000, 0.9238795325112867385, 1.000000000000000000, 0.9238795325112867385, 1.000000000000000000, 0.9238795325112867385, 1.000000000000000000, 0.9238795325112867385, 1.000000000000000000, 0.9238795325112867385, 1.000000000000000000, 0.9238795325112867385, 1.000000000000000000, 0.9238795325112867385, 1.000000000000000000, 0.9238795325112867385, 1.000000000000000000, 0.9238795325112867385, 1.000000000000000000, 0.9238795325112867385, 1.000000000000000000, 0.9238795325112867385, 1.000000000000000000, 0.9238795325112867385, 1.000000000000000000, 0.9238795325112867385, 1.000000000000000000, 0.9238795325112867385, 1.000000000000000000, 0.9238795325112867385, 1.000000000000000000, 0.9238795325112867385, 1.000000000000000000, 0.9238795325112867385, 1.000000000000000000, 0.9238795325112867385, 1.000000000000000000, 0.9238795325112867385, 1.000000000000000000, 0.9238795325112867385, 1.000000000000000000, 0.9238795325112867385, 1.000000000000000000, 0.9238795325112867385, 1.000000000000000000, 0.9238795325112867385, 1.000000000000000000, 0.9238795325112867385, 1.000000000000000000, 0.9238795325112867385, 1.000000000000000000, 0.9238795325112867385, 1.000000000000000000, 0.9238795325112867385, 1.000000000000000000, 0.9238795325112867385, 1.000000000000000000, 0.9462258450566536361, 0.9684275698016389100) ) ) 
 REPRESENTATION_ITEM ( '' )  SURFACE ( )  );
#9399=CARTESIAN_POINT ( 'NONE',  ( 9.295050272127046043, 37.27929687608394005, -9.295050272127046043 ) ) ;
#9408=FACE_OUTER_BOUND ( 'NONE', #14008, .T. ) ;
#9411=CARTESIAN_POINT ( 'NONE',  ( -13.57481594606304576, 33.06249999999999289, 0.000000000000000000 ) ) ;
#9428=PRODUCT_DEFINITION ( 'UNKNOWN', '', #27259, #20902 ) ;
#9432=CARTESIAN_POINT ( 'NONE',  ( -9.295050272127044266, 37.47773437608393010, 9.295050272127047819 ) ) ;
#9481=CARTESIAN_POINT ( 'NONE',  ( -9.295050272127044266, 35.89023437608393152, 9.295050272127047819 ) ) ;
#9508=FACE_OUTER_BOUND ( 'NONE', #23259, .T. ) ;
#9518=CARTESIAN_POINT ( 'NONE',  ( 9.598844408820459861, 32.56640625000000000, 9.598844408820456309 ) ) ;
#9519=CARTESIAN_POINT ( 'NONE',  ( -3.420220812170877700, 35.99999999999999289, -13.02105590829194348 ) ) ;
#9520=CARTESIAN_POINT ( 'NONE',  ( 9.295050272127047819, 33.90585937608393863, 9.295050272127046043 ) ) ;
#9522=CARTESIAN_POINT ( 'NONE',  ( -9.295050272127046043, 34.89804687608393152, -9.295050272127046043 ) ) ;
#9523=CARTESIAN_POINT ( 'NONE',  ( -5.622872871577873077, 34.60039062716786873, -13.57481594606304753 ) ) ;
#9547=CARTESIAN_POINT ( 'NONE',  ( -5.444914386472297529, 37.42812500108394147, -13.14518615778179900 ) ) ;
#9577=CARTESIAN_POINT ( 'NONE',  ( -9.295050272127046043, 36.48554687608393721, -9.295050272127046043 ) ) ;
#9626=CARTESIAN_POINT ( 'NONE',  ( -3.061616997868383831E-15, 0.000000000000000000, -25.00000000000000711 ) ) ;
#9644=CARTESIAN_POINT ( 'NONE',  ( 5.444914386472302859, 33.06250000108393294, 13.14518615778179189 ) ) ;
#9654=CARTESIAN_POINT ( 'NONE',  ( -13.57481594606304753, 35.39414062499999147, -5.622872871577872189 ) ) ;
#9656=CARTESIAN_POINT ( 'NONE',  ( 2.493653234604083739E-15, 35.64218749999999147, 13.57481594606304576 ) ) ;
#9658=CARTESIAN_POINT ( 'NONE',  ( -9.295050272127044266, 34.50117187608393721, 9.295050272127047819 ) ) ;
#9660=CARTESIAN_POINT ( 'NONE',  ( -13.14518615778179722, 34.94765625108394147, -5.444914386472297529 ) ) ;
#9661=CARTESIAN_POINT ( 'NONE',  ( 13.57481594606304576, 36.73359375216787015, -1.662435489736055892E-15 ) ) ;
#9683=ORIENTED_EDGE ( 'NONE', *, *, #10318, .T. ) ;
#9690=CARTESIAN_POINT ( 'NONE',  ( 5.444914386472302859, 37.82500000108392868, 13.14518615778179189 ) ) ;
#9700=CARTESIAN_POINT ( 'NONE',  ( -8.312177448680279460E-16, 32.86406249999999574, -13.57481594606304576 ) ) ;
#9710=ORIENTED_EDGE ( 'NONE', *, *, #19439, .T. ) ;
#9720=CARTESIAN_POINT ( 'NONE',  ( -8.049105076161786076E-16, 37.18007812608393436, -13.14518615778179544 ) ) ;
#9781=VERTEX_POINT ( 'NONE', #12272 ) ;
#9784=CARTESIAN_POINT ( 'NONE',  ( -9.295050272127046043, 33.50898437608393010, -9.295050272127046043 ) ) ;
#9797=CARTESIAN_POINT ( 'NONE',  ( -9.598844408820454532, 34.74921874999999716, 9.598844408820459861 ) ) ;
#9799=CARTESIAN_POINT ( 'NONE',  ( 5.444914386472302859, 34.65000000108393863, 13.14518615778179189 ) ) ;
#9802=CARTESIAN_POINT ( 'NONE',  ( 13.57481594606304576, 35.93984375216787441, -1.662435489736055892E-15 ) ) ;
#9807=DIRECTION ( 'NONE',  ( 0.000000000000000000, 0.000000000000000000, 1.000000000000000000 ) ) ;
#9824=ORIENTED_EDGE ( 'NONE', *, *, #8760, .T. ) ;
#9825=CARTESIAN_POINT ( 'NONE',  ( -13.14518615778179544, 32.02070312608393010, 0.000000000000000000 ) ) ;
#9859=CARTESIAN_POINT ( 'NONE',  ( -5.444914386472297529, 35.64218750108392442, -13.14518615778179900 ) ) ;
#9862=DIRECTION ( 'NONE',  ( 0.000000000000000000, 0.000000000000000000, 1.000000000000000000 ) ) ;
#9880=CARTESIAN_POINT ( 'NONE',  ( -9.598844408820454532, 33.16171874999999858, 9.598844408820459861 ) ) ;
#9881=ORIENTED_EDGE ( 'NONE', *, *, #17078, .T. ) ;
#9886=ORIENTED_EDGE ( 'NONE', *, *, #14686, .F. ) ;
#9901=CARTESIAN_POINT ( 'NONE',  ( 13.14518615778179900, 40.40468750108393436, -5.444914386472297529 ) ) ;
#9902=DIRECTION ( 'NONE',  ( 1.224646799147353454E-16, 0.000000000000000000, -1.000000000000000000 ) ) ;
#9915=CARTESIAN_POINT ( 'NONE',  ( 9.295050272127047819, 32.31835937608393294, 9.295050272127046043 ) ) ;
#9927=CARTESIAN_POINT ( 'NONE',  ( -9.598844408820458085, 35.34453124999998863, -9.598844408820458085 ) ) ;
#9930=CARTESIAN_POINT ( 'NONE',  ( 2.414731522848535132E-15, 32.21914062608393436, 13.14518615778179544 ) ) ;
#9933=CARTESIAN_POINT ( 'NONE',  ( -5.622872871577873077, 33.80664062716786589, -13.57481594606304753 ) ) ;
#9959=CARTESIAN_POINT ( 'NONE',  ( 13.14518615778179900, 32.46718750108393436, -5.444914386472297529 ) ) ;
#9966=DIRECTION ( 'NONE',  ( 0.000000000000000000, 0.000000000000000000, -1.000000000000000000 ) ) ;
#9991=CARTESIAN_POINT ( 'NONE',  ( -8.049105076161786076E-16, 34.79882812608393294, -13.14518615778179544 ) ) ;
#10004=CARTESIAN_POINT ( 'NONE',  ( -13.14518615778179189, 37.42812500108393436, 5.444914386472304635 ) ) ;
#10015=AXIS2_PLACEMENT_3D ( 'NONE', #3266, #11933, #9807 ) ;
#10023=CARTESIAN_POINT ( 'NONE',  ( 0.000000000000000000, 10.00000000000000000, 0.000000000000000000 ) ) ;
#10028=DIRECTION ( 'NONE',  ( -0.000000000000000000, -1.000000000000000000, -0.000000000000000000 ) ) ;
#10037=CARTESIAN_POINT ( 'NONE',  ( 5.444914386472302859, 39.41250000108393436, 13.14518615778179189 ) ) ;
#10067=CARTESIAN_POINT ( 'NONE',  ( 13.57481594606304753, 40.65273437499998721, -5.622872871577873077 ) ) ;
#10069=CARTESIAN_POINT ( 'NONE',  ( -13.57481594606304576, 31.62382812716787228, 5.622872871577880183 ) ) ;
#10079=VERTEX_POINT ( 'NONE', #21208 ) ;
#10090=CARTESIAN_POINT ( 'NONE',  ( -5.444914386472297529, 34.25312500108393010, -13.14518615778179900 ) ) ;
#10101=SHAPE_DEFINITION_REPRESENTATION ( #13995, #9145 ) ;
#10107=CARTESIAN_POINT ( 'NONE',  ( -12.73839015785546813, 35.99999999999998579, 3.273369733618573196 ) ) ;
#10120=CARTESIAN_POINT ( 'NONE',  ( -9.295050272127046043, 34.89804687608393152, -9.295050272127046043 ) ) ;
#10134=CARTESIAN_POINT ( 'NONE',  ( -9.295050272127044266, 34.30273437608393294, 9.295050272127047819 ) ) ;
#10197=CARTESIAN_POINT ( 'NONE',  ( -13.57481594606304576, 32.31835937499999289, 5.622872871577880183 ) ) ;
#10201=CARTESIAN_POINT ( 'NONE',  ( 13.57481594606304753, 39.06523437499998863, -5.622872871577873077 ) ) ;
#10202=CARTESIAN_POINT ( 'NONE',  ( 2.414731522848535132E-15, 33.60820312608392868, 13.14518615778179544 ) ) ;
#10204=CARTESIAN_POINT ( 'NONE',  ( -8.312177448680279460E-16, 32.16953125216787157, -13.57481594606304576 ) ) ;
#10225=ORIENTED_EDGE ( 'NONE', *, *, #2205, .T. ) ;
#10226=CARTESIAN_POINT ( 'NONE',  ( 6.944426393311538881, 31.75150625057403175, -11.16113171639042356 ) ) ;
#10232=CARTESIAN_POINT ( 'NONE',  ( 0.000000000000000000, 31.00000000000000000, 0.000000000000000000 ) ) ;
#10241=AXIS2_PLACEMENT_3D ( 'NONE', #23336, #25744, #23474 ) ;
#10255=CARTESIAN_POINT ( 'NONE',  ( 9.598844408820456309, 32.76484374999999716, -9.598844408820458085 ) ) ;
#10259=CARTESIAN_POINT ( 'NONE',  ( 5.444914386472302859, 33.65781250108393152, 13.14518615778179189 ) ) ;
#10275=CARTESIAN_POINT ( 'NONE',  ( 13.14518615778179900, 32.16953125108393152, 5.444914386472293977 ) ) ;
#10278=ORIENTED_EDGE ( 'NONE', *, *, #19932, .T. ) ;
#10305=CARTESIAN_POINT ( 'NONE',  ( 2.493653234604083739E-15, 31.77265625216787370, 13.57481594606304576 ) ) ;
#10318=EDGE_CURVE ( 'NONE', #22337, #9781, #8761, .T. ) ;
#10340=CARTESIAN_POINT ( 'NONE',  ( -13.14518615778179544, 32.02070312608393010, 0.000000000000000000 ) ) ;
#10342=CARTESIAN_POINT ( 'NONE',  ( 5.444914386472302859, 32.86406250108392868, 13.14518615778179189 ) ) ;
#10343=CARTESIAN_POINT ( 'NONE',  ( 5.622872871577871301, 32.91367187716787157, -13.57481594606304753 ) ) ;
#10371=ADVANCED_FACE ( 'NONE', ( #22762 ), #26899, .T. ) ;
#10399=VERTEX_POINT ( 'NONE', #27186 ) ;
#10405=CARTESIAN_POINT ( 'NONE',  ( -5.444914386472297529, 33.26093750108393721, -13.14518615778179900 ) ) ;
#10422=CARTESIAN_POINT ( 'NONE',  ( -8.049105076161786076E-16, 31.62382812608393579, -13.14518615778179544 ) ) ;
#10435=DIRECTION ( 'NONE',  ( 0.000000000000000000, 1.000000000000000000, 0.000000000000000000 ) ) ;
#10437=ORIENTED_EDGE ( 'NONE', *, *, #12599, .F. ) ;
#10478=( NAMED_UNIT ( * ) SI_UNIT ( $, .STERADIAN. ) SOLID_ANGLE_UNIT ( ) );
#10484=CARTESIAN_POINT ( 'NONE',  ( 13.57481594606304753, 39.85898437499999858, -5.622872871577873077 ) ) ;
#10486=CARTESIAN_POINT ( 'NONE',  ( -13.57481594606304576, 33.16171875216787868, 0.000000000000000000 ) ) ;
#10504=AXIS2_PLACEMENT_3D ( 'NONE', #12126, #25404, #14555 ) ;
#10539=ORIENTED_EDGE ( 'NONE', *, *, #28153, .F. ) ;
#10540=( BOUNDED_SURFACE ( )  B_SPLINE_SURFACE ( 1, 2, ( 
 ( #15907, #9364, #20068, #2955, #5103, #14058, #11772, #9227, #20497, #15774, #15636, #24626, #22489, #26773, #1120, #26917, #22348, #16201, #13628, #27058, #3247, #18058, #17920, #26631, #18350, #16055, #7078, #20352, #13766, #7217, #24480, #837, #980, #7361, #4966, #24764, #2819, #13483, #11487, #17782, #26485, #20203, #7508, #24337, #24907, #5388, #22778, #11914, #20636, #6940, #4823, #22205, #690, #24777, #16069, #24918, #13922, #9241, #2967, #7669, #5258, #13499, #17933, #26931, #20511, #5115, #11788, #18073, #11358, #26643, #22650, #993, #9661, #11642, #7232, #4838, #7375, #7091, #2698, #15790, #16217, #3120, #20082, #18364, #22219, #13644, #16361, #27071, #9802, #7522, #24493, #18508, #5402, #20650, #14072, #22792, #3261, #2833, #15923, #4978, #11928, #22359, #1134, #20366, #851, #27214, #559, #11501, #20218, #703, #9376, #26787, #24641, #13780, #22502, #9523, #18223, #8218, #12199, #14622, #12063, #5548, #14213, #18648, #25333, #16908, #21342, #20788, #7811, #25062, #18781, #9933, #22931, #8081, #25606, #1269, #27759, #25476, #6090, #5819, #16776, #27353, #16503, #3392, #10486, #19194, #14489, #12345, #23206, #10343, #12474, #19050, #14757, #23477, #25197, #3681, #21063, #1821, #21201, #5683, #1684, #23064, #14349, #1551, #10204, #18914, #8357, #5955, #1410, #3957, #20927, #12617, #27897, #16641, #3542, #10069, #27488, #23340, #7945, #27623, #3814, #8643, #10626 ),
 ( #12757, #10762, #380, #25747, #8501, #26026, #23617, #17332, #21764, #15319, #17608, #4371, #21908, #2383, #6497, #8920, #11041, #25893, #24033, #21478, #17466, #17043, #6363, #26316, #12888, #10903, #1957, #2094, #28172, #19896, #6229, #2241, #4094, #19750, #13027, #15462, #19331, #233, #19473, #15173, #97, #26168, #14896, #6635, #28034, #4512, #23752, #13169, #23892, #15035, #8778, #19612, #21618, #6777, #24177, #4654, #17186, #4230, #13315, #22041, #2516, #11178, #24603, #10004, #16570, #17897, #7190, #667, #2932, #26606, #12271, #16028, #22326, #15609, #2661, #26892, #25125, #5612, #15888, #11464, #9064, #11602, #22181, #6916, #11322, #20858, #20325, #24311, #7339, #17759, #7052, #20997, #813, #14421, #9481, #20043, #23136, #18182, #25261, #14278, #3466, #7876, #15751, #20183, #522, #18713, #9203, #1340, #5081, #13743, #12132, #22996, #27413, #5752, #24454, #4940, #3612, #9340, #26462, #4797, #18035, #13604, #13455, #2797, #26748, #22467, #10134, #18846, #23277, #1756, #21556, #25965, #25410, #12412, #1478, #23411, #14562, #8289, #6438, #5892, #27555, #3750, #15107, #25822, #6027, #21132, #4169, #14973, #1897, #27694, #4308, #21419, #12965, #6296, #10699, #8012, #16713, #14691, #14828, #6162, #17264, #18984, #12829, #23692, #3885, #21273, #1617, #27835, #23552, #10275, #2030, #19272, #8156, #27971, #16848, #25547, #12546, #19405, #16981, #23828, #10422, #4029, #28110 ) ),
 .UNSPECIFIED., .F., .F., .F. ) 
 B_SPLINE_SURFACE_WITH_KNOTS ( ( 2, 2 ),
 ( 3, 2, 2, 2, 2, 2, 2, 2, 2, 2, 2, 2, 2, 2, 2, 2, 2, 2, 2, 2, 2, 2, 2, 2, 2, 2, 2, 2, 2, 2, 2, 2, 2, 2, 2, 2, 2, 2, 2, 2, 2, 2, 2, 2, 2, 2, 2, 2, 2, 2, 2, 2, 2, 2, 2, 2, 2, 2, 2, 2, 2, 2, 2, 2, 2, 2, 2, 2, 2, 2, 2, 2, 2, 2, 2, 2, 2, 2, 2, 2, 2, 2, 2, 2, 2, 2, 2, 2, 2, 2, 2, 3 ),
 ( 0.000000000000000000, 1.000000000000000000 ),
 ( 0.000000000000000000, 0.01041666666666666609, 0.02083333333333333218, 0.03125000000000000000, 0.04166666666666666435, 0.05208333333333333565, 0.06250000000000000000, 0.07291666666666667129, 0.08333333333333332871, 0.09375000000000000000, 0.1041666666666666713, 0.1145833333333333287, 0.1250000000000000000, 0.1354166666666666574, 0.1458333333333333426, 0.1562500000000000000, 0.1666666666666666574, 0.1770833333333333426, 0.1875000000000000000, 0.1979166666666666574, 0.2083333333333333426, 0.2187500000000000000, 0.2291666666666666574, 0.2395833333333333426, 0.2500000000000000000, 0.2604166666666666852, 0.2708333333333333148, 0.2812500000000000000, 0.2916666666666666852, 0.3020833333333333148, 0.3125000000000000000, 0.3229166666666666852, 0.3333333333333333148, 0.3437500000000000000, 0.3541666666666666852, 0.3645833333333333148, 0.3750000000000000000, 0.3854166666666666852, 0.3958333333333333148, 0.4062500000000000000, 0.4166666666666666852, 0.4270833333333333148, 0.4375000000000000000, 0.4479166666666666852, 0.4583333333333333148, 0.4687500000000000000, 0.4791666666666666852, 0.4895833333333333148, 0.5000000000000000000, 0.5104166666666666297, 0.5208333333333333703, 0.5312500000000000000, 0.5416666666666666297, 0.5520833333333333703, 0.5625000000000000000, 0.5729166666666666297, 0.5833333333333333703, 0.5937500000000000000, 0.6041666666666666297, 0.6145833333333333703, 0.6250000000000000000, 0.6354166666666666297, 0.6458333333333333703, 0.6562500000000000000, 0.6666666666666666297, 0.6770833333333333703, 0.6875000000000000000, 0.6979166666666666297, 0.7083333333333333703, 0.7187500000000000000, 0.7291666666666666297, 0.7395833333333333703, 0.7500000000000000000, 0.7604166666666666297, 0.7708333333333333703, 0.7812500000000000000, 0.7916666666666666297, 0.8020833333333333703, 0.8125000000000000000, 0.8229166666666666297, 0.8333333333333333703, 0.8437500000000000000, 0.8541666666666666297, 0.8645833333333333703, 0.8750000000000000000, 0.8854166666666666297, 0.8958333333333333703, 0.9062500000000000000, 0.9166666666666666297, 0.9270833333333333703, 0.9375000000000000000, 0.9448586970929392370 ),
 .UNSPECIFIED. ) 
 GEOMETRIC_REPRESENTATION_ITEM ( )  RATIONAL_B_SPLINE_SURFACE ( (
 ( 1.000000000000000000, 0.9238795325112867385, 1.000000000000000000, 0.9238795325112867385, 1.000000000000000000, 0.9238795325112867385, 1.000000000000000000, 0.9238795325112867385, 1.000000000000000000, 0.9238795325112867385, 1.000000000000000000, 0.9238795325112867385, 1.000000000000000000, 0.9238795325112867385, 1.000000000000000000, 0.9238795325112867385, 1.000000000000000000, 0.9238795325112867385, 1.000000000000000000, 0.9238795325112867385, 1.000000000000000000, 0.9238795325112867385, 1.000000000000000000, 0.9238795325112867385, 1.000000000000000000, 0.9238795325112867385, 1.000000000000000000, 0.9238795325112867385, 1.000000000000000000, 0.9238795325112867385, 1.000000000000000000, 0.9238795325112867385, 1.000000000000000000, 0.9238795325112867385, 1.000000000000000000, 0.9238795325112867385, 1.000000000000000000, 0.9238795325112867385, 1.000000000000000000, 0.9238795325112867385, 1.000000000000000000, 0.9238795325112867385, 1.000000000000000000, 0.9238795325112867385, 1.000000000000000000, 0.9238795325112867385, 1.000000000000000000, 0.9238795325112867385, 1.000000000000000000, 0.9238795325112867385, 1.000000000000000000, 0.9238795325112867385, 1.000000000000000000, 0.9238795325112867385, 1.000000000000000000, 0.9238795325112867385, 1.000000000000000000, 0.9238795325112867385, 1.000000000000000000, 0.9238795325112867385, 1.000000000000000000, 0.9238795325112867385, 1.000000000000000000, 0.9238795325112867385, 1.000000000000000000, 0.9238795325112867385, 1.000000000000000000, 0.9238795325112867385, 1.000000000000000000, 0.9238795325112867385, 1.000000000000000000, 0.9238795325112867385, 1.000000000000000000, 0.9238795325112867385, 1.000000000000000000, 0.9238795325112867385, 1.000000000000000000, 0.9238795325112867385, 1.000000000000000000, 0.9238795325112867385, 1.000000000000000000, 0.9238795325112867385, 1.000000000000000000, 0.9238795325112867385, 1.000000000000000000, 0.9238795325112867385, 1.000000000000000000, 0.9238795325112867385, 1.000000000000000000, 0.9238795325112867385, 1.000000000000000000, 0.9238795325112867385, 1.000000000000000000, 0.9238795325112867385, 1.000000000000000000, 0.9238795325112867385, 1.000000000000000000, 0.9238795325112867385, 1.000000000000000000, 0.9238795325112867385, 1.000000000000000000, 0.9238795325112867385, 1.000000000000000000, 0.9238795325112867385, 1.000000000000000000, 0.9238795325112867385, 1.000000000000000000, 0.9238795325112867385, 1.000000000000000000, 0.9238795325112867385, 1.000000000000000000, 0.9238795325112867385, 1.000000000000000000, 0.9238795325112867385, 1.000000000000000000, 0.9238795325112867385, 1.000000000000000000, 0.9238795325112867385, 1.000000000000000000, 0.9238795325112867385, 1.000000000000000000, 0.9238795325112867385, 1.000000000000000000, 0.9238795325112867385, 1.000000000000000000, 0.9238795325112867385, 1.000000000000000000, 0.9238795325112867385, 1.000000000000000000, 0.9238795325112867385, 1.000000000000000000, 0.9238795325112867385, 1.000000000000000000, 0.9238795325112867385, 1.000000000000000000, 0.9238795325112867385, 1.000000000000000000, 0.9238795325112867385, 1.000000000000000000, 0.9238795325112867385, 1.000000000000000000, 0.9238795325112867385, 1.000000000000000000, 0.9238795325112867385, 1.000000000000000000, 0.9238795325112867385, 1.000000000000000000, 0.9238795325112867385, 1.000000000000000000, 0.9238795325112867385, 1.000000000000000000, 0.9238795325112867385, 1.000000000000000000, 0.9238795325112867385, 1.000000000000000000, 0.9238795325112867385, 1.000000000000000000, 0.9238795325112867385, 1.000000000000000000, 0.9238795325112867385, 1.000000000000000000, 0.9238795325112867385, 1.000000000000000000, 0.9238795325112867385, 1.000000000000000000, 0.9238795325112867385, 1.000000000000000000, 0.9238795325112867385, 1.000000000000000000, 0.9238795325112867385, 1.000000000000000000, 0.9238795325112867385, 1.000000000000000000, 0.9238795325112867385, 1.000000000000000000, 0.9238795325112867385, 1.000000000000000000, 0.9238795325112867385, 1.000000000000000000, 0.9238795325112867385, 1.000000000000000000, 0.9462258435690522607, 0.9684275710300105366),
 ( 1.000000000000000000, 0.9238795325112867385, 1.000000000000000000, 0.9238795325112867385, 1.000000000000000000, 0.9238795325112867385, 1.000000000000000000, 0.9238795325112867385, 1.000000000000000000, 0.9238795325112867385, 1.000000000000000000, 0.9238795325112867385, 1.000000000000000000, 0.9238795325112867385, 1.000000000000000000, 0.9238795325112867385, 1.000000000000000000, 0.9238795325112867385, 1.000000000000000000, 0.9238795325112867385, 1.000000000000000000, 0.9238795325112867385, 1.000000000000000000, 0.9238795325112867385, 1.000000000000000000, 0.9238795325112867385, 1.000000000000000000, 0.9238795325112867385, 1.000000000000000000, 0.9238795325112867385, 1.000000000000000000, 0.9238795325112867385, 1.000000000000000000, 0.9238795325112867385, 1.000000000000000000, 0.9238795325112867385, 1.000000000000000000, 0.9238795325112867385, 1.000000000000000000, 0.9238795325112867385, 1.000000000000000000, 0.9238795325112867385, 1.000000000000000000, 0.9238795325112867385, 1.000000000000000000, 0.9238795325112867385, 1.000000000000000000, 0.9238795325112867385, 1.000000000000000000, 0.9238795325112867385, 1.000000000000000000, 0.9238795325112867385, 1.000000000000000000, 0.9238795325112867385, 1.000000000000000000, 0.9238795325112867385, 1.000000000000000000, 0.9238795325112867385, 1.000000000000000000, 0.9238795325112867385, 1.000000000000000000, 0.9238795325112867385, 1.000000000000000000, 0.9238795325112867385, 1.000000000000000000, 0.9238795325112867385, 1.000000000000000000, 0.9238795325112867385, 1.000000000000000000, 0.9238795325112867385, 1.000000000000000000, 0.9238795325112867385, 1.000000000000000000, 0.9238795325112867385, 1.000000000000000000, 0.9238795325112867385, 1.000000000000000000, 0.9238795325112867385, 1.000000000000000000, 0.9238795325112867385, 1.000000000000000000, 0.9238795325112867385, 1.000000000000000000, 0.9238795325112867385, 1.000000000000000000, 0.9238795325112867385, 1.000000000000000000, 0.9238795325112867385, 1.000000000000000000, 0.9238795325112867385, 1.000000000000000000, 0.9238795325112867385, 1.000000000000000000, 0.9238795325112867385, 1.000000000000000000, 0.9238795325112867385, 1.000000000000000000, 0.9238795325112867385, 1.000000000000000000, 0.9238795325112867385, 1.000000000000000000, 0.9238795325112867385, 1.000000000000000000, 0.9238795325112867385, 1.000000000000000000, 0.9238795325112867385, 1.000000000000000000, 0.9238795325112867385, 1.000000000000000000, 0.9238795325112867385, 1.000000000000000000, 0.9238795325112867385, 1.000000000000000000, 0.9238795325112867385, 1.000000000000000000, 0.9238795325112867385, 1.000000000000000000, 0.9238795325112867385, 1.000000000000000000, 0.9238795325112867385, 1.000000000000000000, 0.9238795325112867385, 1.000000000000000000, 0.9238795325112867385, 1.000000000000000000, 0.9238795325112867385, 1.000000000000000000, 0.9238795325112867385, 1.000000000000000000, 0.9238795325112867385, 1.000000000000000000, 0.9238795325112867385, 1.000000000000000000, 0.9238795325112867385, 1.000000000000000000, 0.9238795325112867385, 1.000000000000000000, 0.9238795325112867385, 1.000000000000000000, 0.9238795325112867385, 1.000000000000000000, 0.9238795325112867385, 1.000000000000000000, 0.9238795325112867385, 1.000000000000000000, 0.9238795325112867385, 1.000000000000000000, 0.9238795325112867385, 1.000000000000000000, 0.9238795325112867385, 1.000000000000000000, 0.9238795325112867385, 1.000000000000000000, 0.9238795325112867385, 1.000000000000000000, 0.9238795325112867385, 1.000000000000000000, 0.9238795325112867385, 1.000000000000000000, 0.9238795325112867385, 1.000000000000000000, 0.9238795325112867385, 1.000000000000000000, 0.9238795325112867385, 1.000000000000000000, 0.9238795325112867385, 1.000000000000000000, 0.9238795325112867385, 1.000000000000000000, 0.9238795325112867385, 1.000000000000000000, 0.9238795325112867385, 1.000000000000000000, 0.9238795325112867385, 1.000000000000000000, 0.9238795325112867385, 1.000000000000000000, 0.9238795325112867385, 1.000000000000000000, 0.9238795325112867385, 1.000000000000000000, 0.9462258435690522607, 0.9684275710300105366) ) ) 
 REPRESENTATION_ITEM ( '' )  SURFACE ( )  );
#10542=VERTEX_POINT ( 'NONE', #23174 ) ;
#10543=CARTESIAN_POINT ( 'NONE',  ( -9.295050272127046043, 35.89023437608393152, -9.295050272127046043 ) ) ;
#10544=CARTESIAN_POINT ( 'NONE',  ( 5.444914386472297529, 33.95546875108393436, -13.14518615778179900 ) ) ;
#10565=ADVANCED_FACE ( 'NONE', ( #3785 ), #26000, .T. ) ;
#10625=CARTESIAN_POINT ( 'NONE',  ( -13.14518615778179722, 31.77265625108393365, -5.444914386472297529 ) ) ;
#10626=CARTESIAN_POINT ( 'NONE',  ( 7.171391395016640580, 31.30502190640808990, -11.52591746582321974 ) ) ;
#10644=CARTESIAN_POINT ( 'NONE',  ( 13.39333672780506035, 36.00000000000000000, -2.034633736484789068 ) ) ;
#10654=CARTESIAN_POINT ( 'NONE',  ( 9.295050272127046043, 37.27929687608394005, -9.295050272127046043 ) ) ;
#10664=CARTESIAN_POINT ( 'NONE',  ( -9.115657261794327226, 36.00000000000000711, 9.510219181138872102 ) ) ;
#10679=CARTESIAN_POINT ( 'NONE',  ( 9.295050272127047819, 35.49335937608393721, 9.295050272127046043 ) ) ;
#10680=CARTESIAN_POINT ( 'NONE',  ( -13.14518615778179544, 38.37070312608393152, 0.000000000000000000 ) ) ;
#10697=CIRCLE ( 'NONE', #19828, 23.00000000000001421 ) ;
#10699=CARTESIAN_POINT ( 'NONE',  ( 9.295050272127047819, 32.91367187608393152, 9.295050272127046043 ) ) ;
#10716=CARTESIAN_POINT ( 'NONE',  ( 9.295050272127047819, 38.46992187608393010, 9.295050272127046043 ) ) ;
#10734=DIRECTION ( 'NONE',  ( 0.000000000000000000, 0.000000000000000000, 1.000000000000000000 ) ) ;
#10751=CARTESIAN_POINT ( 'NONE',  ( -9.295050272127044266, 34.50117187608393721, 9.295050272127047819 ) ) ;
#10762=CARTESIAN_POINT ( 'NONE',  ( -13.14518615778179900, 40.50390625108394005, -5.444914386472297529 ) ) ;
#10790=CARTESIAN_POINT ( 'NONE',  ( 5.622872871577878406, 38.07304687499998863, 13.57481594606304576 ) ) ;
#10792=CARTESIAN_POINT ( 'NONE',  ( 13.14518615778179900, 36.33671875108394289, 5.444914386472293977 ) ) ;
#10815=CARTESIAN_POINT ( 'NONE',  ( -9.295050272127044266, 35.29492187608393294, 9.295050272127047819 ) ) ;
#10816=CARTESIAN_POINT ( 'NONE',  ( -5.444914386472297529, 31.67343750108393863, -13.14518615778179900 ) ) ;
#10822=EDGE_LOOP ( 'NONE', ( #11460, #19662, #1217, #15670 ) ) ;
#10826=LINE ( 'NONE', #12956, #12744 ) ;
#10851=CARTESIAN_POINT ( 'NONE',  ( -9.295050272127046043, 40.45429687608393721, -9.295050272127046043 ) ) ;
#10867=EDGE_CURVE ( 'NONE', #11809, #25304, #1139, .T. ) ;
#10903=CARTESIAN_POINT ( 'NONE',  ( 13.14518615778179900, 39.31328125108392868, 5.444914386472293977 ) ) ;
#10922=CARTESIAN_POINT ( 'NONE',  ( 6.351932228772031230, 36.00000000000000000, 11.61660627739472140 ) ) ;
#10931=CARTESIAN_POINT ( 'NONE',  ( 13.57481594606304931, 36.58476562499999574, 5.622872871577869525 ) ) ;
#10933=CARTESIAN_POINT ( 'NONE',  ( -13.14518615778179189, 37.62656250108393863, 5.444914386472304635 ) ) ;
#10958=ORIENTED_EDGE ( 'NONE', *, *, #21043, .T. ) ;
#10960=CARTESIAN_POINT ( 'NONE',  ( -9.295050272127044266, 39.26367187608393294, 9.295050272127047819 ) ) ;
#10990=CARTESIAN_POINT ( 'NONE',  ( 9.295050272127046043, 39.46210937608393010, -9.295050272127046043 ) ) ;
#10996=CARTESIAN_POINT ( 'NONE',  ( -13.57481594606304576, 34.74921875216787726, 0.000000000000000000 ) ) ;
#11026=FACE_OUTER_BOUND ( 'NONE', #14057, .T. ) ;
#11028=DIRECTION ( 'NONE',  ( 0.000000000000000000, 0.000000000000000000, 1.000000000000000000 ) ) ;
#11034=FILL_AREA_STYLE_COLOUR ( '', #17710 ) ;
#11040=EDGE_CURVE ( 'NONE', #8271, #20304, #27357, .T. ) ;
#11041=CARTESIAN_POINT ( 'NONE',  ( -13.14518615778179544, 39.75976562608393294, 0.000000000000000000 ) ) ;
#11047=ADVANCED_BREP_SHAPE_REPRESENTATION ( '', ( #16871, #26844 ), #17253 ) ;
#11059=CARTESIAN_POINT ( 'NONE',  ( 1.685511649082876318, 35.99999999999997868, 13.05727741351675775 ) ) ;
#11072=CARTESIAN_POINT ( 'NONE',  ( -5.622872871577688336, 32.21914062716787441, -13.57481594606323050 ) ) ;
#11073=CARTESIAN_POINT ( 'NONE',  ( 2.493653234604083739E-15, 38.81718749999999574, 13.57481594606304576 ) ) ;
#11074=CARTESIAN_POINT ( 'NONE',  ( 9.295050272127046043, 36.48554687608393721, -9.295050272127046043 ) ) ;
#11100=CARTESIAN_POINT ( 'NONE',  ( -8.049105076161786076E-16, 32.61601562608393579, -13.14518615778179544 ) ) ;
#11101=CARTESIAN_POINT ( 'NONE',  ( -8.049105076161786076E-16, 40.55351562608393579, -13.14518615778179544 ) ) ;
#11109=CARTESIAN_POINT ( 'NONE',  ( -9.598844408820458085, 34.55078124999999289, -9.598844408820458085 ) ) ;
#11111=DIRECTION ( 'NONE',  ( 0.000000000000000000, 0.000000000000000000, 1.000000000000000000 ) ) ;
#11113=CARTESIAN_POINT ( 'NONE',  ( 0.000000000000000000, 31.00000000000000000, -13.57481594606304576 ) ) ;
#11114=DIRECTION ( 'NONE',  ( 0.000000000000000000, 0.000000000000000000, -1.000000000000000000 ) ) ;
#11122=DIRECTION ( 'NONE',  ( 0.000000000000000000, 0.000000000000000000, 1.000000000000000000 ) ) ;
#11178=CARTESIAN_POINT ( 'NONE',  ( -5.444914386472299306, 37.52734375108393294, 13.14518615778179722 ) ) ;
#11194=( BOUNDED_CURVE ( )  B_SPLINE_CURVE ( 2, ( #1374, #23030, #5923, #8187, #5645, #14589, #23168, #3781, #25576 ),
 .UNSPECIFIED., .F., .T. ) 
 B_SPLINE_CURVE_WITH_KNOTS ( ( 3, 2, 2, 2, 3 ),
 ( 0.6041666666666668517, 0.6145833333333334814, 0.6250000000000001110, 0.6354166666666667407, 0.6458333333333333703 ),
 .UNSPECIFIED. ) 
 CURVE ( )  GEOMETRIC_REPRESENTATION_ITEM ( )  RATIONAL_B_SPLINE_CURVE ( ( 0.9999999999999983347, 0.9238795325112884038, 1.000000000000000000, 0.9238795325112867385, 1.000000000000000000, 0.9238795325112867385, 1.000000000000000000, 0.9238795325112867385, 1.000000000000000000 ) ) 
 REPRESENTATION_ITEM ( '' )  );
#11211=CARTESIAN_POINT ( 'NONE',  ( -5.622872871577873077, 36.08867187500000284, -13.57481594606304753 ) ) ;
#11214=CARTESIAN_POINT ( 'NONE',  ( 13.14518615778179544, 37.18007812608393436, -1.609821015232357215E-15 ) ) ;
#11223=EDGE_LOOP ( 'NONE', ( #6894, #399, #10278, #21614 ) ) ;
#11230=CARTESIAN_POINT ( 'NONE',  ( 9.598844408820456309, 35.14609374999999858, -9.598844408820458085 ) ) ;
#11238=DIRECTION ( 'NONE',  ( 1.224646799147353454E-16, 0.000000000000000000, -1.000000000000000000 ) ) ;
#11242=CARTESIAN_POINT ( 'NONE',  ( -13.14518615778179544, 35.98945312608393721, 0.000000000000000000 ) ) ;
#11266=CARTESIAN_POINT ( 'NONE',  ( 1.417506129906585201E-15, 36.00000000000000000, 11.57481594606304576 ) ) ;
#11274=CARTESIAN_POINT ( 'NONE',  ( 9.295050272127046043, 40.25585937608393294, -9.295050272127046043 ) ) ;
#11322=CARTESIAN_POINT ( 'NONE',  ( -8.049105076161786076E-16, 36.38632812608393152, -13.14518615778179544 ) ) ;
#11325=( BOUNDED_CURVE ( )  B_SPLINE_CURVE ( 2, ( #7231, #24776, #22357, #7374, #18647, #20217, #24639, #5546, #15789, #18071, #1133, #27352, #992, #14210, #13921, #11641, #4977, #18507, #11786, #26786, #702, #5114, #20509, #9660, #9522, #5257, #22930, #3391, #18221, #9375, #22649, #13643, #18363, #27070, #13779, #16360, #2966, #849, #7521, #11927, #25060, #14621, #12756, #3813, #12344, #12473, #1550, #25475, #14894, #25746, #10202, #14348, #23338, #6228, #21199, #19049, #16500, #19193, #23205, #19330, #25195, #14488, #16907, #1682, #21477, #10342, #21061, #23615, #25332, #23476, #27895, #23063, #1409, #4091, #27757, #1955, #16640, #3541, #7810, #8217, #8356, #18780, #17042, #25604, #6089, #1819, #14756, #10625, #5682, #3955, #12615, #12198, #20926 ),
 .UNSPECIFIED., .F., .F. ) 
 B_SPLINE_CURVE_WITH_KNOTS ( ( 3, 2, 2, 2, 2, 2, 2, 2, 2, 2, 2, 2, 2, 2, 2, 2, 2, 2, 2, 2, 2, 2, 2, 2, 2, 2, 2, 2, 2, 2, 2, 2, 2, 2, 2, 2, 2, 2, 2, 2, 2, 2, 2, 2, 2, 2, 3 ),
 ( 0.4779971559588572227, 0.4791666666666666852, 0.4895833333333333148, 0.5000000000000000000, 0.5104166666666666297, 0.5208333333333333703, 0.5312500000000000000, 0.5416666666666666297, 0.5520833333333333703, 0.5625000000000000000, 0.5729166666666666297, 0.5833333333333333703, 0.5937500000000000000, 0.6041666666666666297, 0.6145833333333333703, 0.6250000000000000000, 0.6354166666666666297, 0.6458333333333333703, 0.6562500000000000000, 0.6666666666666666297, 0.6770833333333333703, 0.6875000000000000000, 0.6979166666666666297, 0.7083333333333333703, 0.7187500000000000000, 0.7291666666666666297, 0.7395833333333333703, 0.7500000000000000000, 0.7604166666666666297, 0.7708333333333333703, 0.7812500000000000000, 0.7916666666666666297, 0.8020833333333333703, 0.8125000000000000000, 0.8229166666666666297, 0.8333333333333333703, 0.8437500000000000000, 0.8541666666666666297, 0.8645833333333333703, 0.8750000000000000000, 0.8854166666666666297, 0.8958333333333333703, 0.9062500000000000000, 0.9166666666666665186, 0.9270833333333333703, 0.9375000000000000000, 0.9448586970929392370 ),
 .UNSPECIFIED. ) 
 CURVE ( )  GEOMETRIC_REPRESENTATION_ITEM ( )  RATIONAL_B_SPLINE_CURVE ( ( 0.9848264816800302857, 0.9914537246260948233, 1.000000000000000000, 0.9238795325112867385, 1.000000000000000000, 0.9238795325112867385, 1.000000000000000000, 0.9238795325112867385, 1.000000000000000000, 0.9238795325112867385, 1.000000000000000000, 0.9238795325112867385, 1.000000000000000000, 0.9238795325112867385, 1.000000000000000000, 0.9238795325112867385, 1.000000000000000000, 0.9238795325112867385, 1.000000000000000000, 0.9238795325112867385, 1.000000000000000000, 0.9238795325112867385, 1.000000000000000000, 0.9238795325112867385, 1.000000000000000000, 0.9238795325112867385, 1.000000000000000000, 0.9238795325112867385, 1.000000000000000000, 0.9238795325112867385, 1.000000000000000000, 0.9238795325112867385, 1.000000000000000000, 0.9238795325112867385, 1.000000000000000000, 0.9238795325112867385, 1.000000000000000000, 0.9238795325112867385, 1.000000000000000000, 0.9238795325112867385, 1.000000000000000000, 0.9238795325112867385, 1.000000000000000000, 0.9238795325112867385, 1.000000000000000000, 0.9238795325112867385, 1.000000000000000000, 0.9238795325112867385, 1.000000000000000000, 0.9238795325112867385, 1.000000000000000000, 0.9238795325112867385, 1.000000000000000000, 0.9238795325112867385, 1.000000000000000000, 0.9238795325112867385, 1.000000000000000000, 0.9238795325112867385, 1.000000000000000000, 0.9238795325112867385, 1.000000000000000000, 0.9238795325112867385, 1.000000000000000000, 0.9238795325112867385, 1.000000000000000000, 0.9238795325112867385, 1.000000000000000000, 0.9238795325112867385, 1.000000000000000000, 0.9238795325112867385, 1.000000000000000000, 0.9238795325112867385, 1.000000000000000000, 0.9238795325112867385, 1.000000000000000000, 0.9238795325112867385, 1.000000000000000000, 0.9238795325112867385, 1.000000000000000000, 0.9238795325112867385, 1.000000000000000000, 0.9238795325112867385, 1.000000000000000000, 0.9238795325112867385, 1.000000000000000000, 0.9238795325112867385, 1.000000000000000000, 0.9238795325112867385, 1.000000000000000000, 0.9238795325112867385, 1.000000000000000000, 0.9462258435690522607, 0.9684275710300105366 ) ) 
 REPRESENTATION_ITEM ( '' )  );
#11345=CARTESIAN_POINT ( 'NONE',  ( 0.000000000000000000, 21.95886589889650509, 0.000000000000000000 ) ) ;
#11353=CARTESIAN_POINT ( 'NONE',  ( -5.622872871577873077, 38.76757812500000000, 13.57481594606304753 ) ) ;
#11354=CARTESIAN_POINT ( 'NONE',  ( -0.1722897647759079331, 36.00000000000000000, -13.51468191220838122 ) ) ;
#11355=CARTESIAN_POINT ( 'NONE',  ( 9.295050272127047819, 35.49335937608393721, 9.295050272127046043 ) ) ;
#11358=CARTESIAN_POINT ( 'NONE',  ( -8.312177448680279460E-16, 36.93203125216787441, -13.57481594606304576 ) ) ;
#11381=DIRECTION ( 'NONE',  ( 0.000000000000000000, 1.000000000000000000, 0.000000000000000000 ) ) ;
#11384=CARTESIAN_POINT ( 'NONE',  ( -8.049105076161786076E-16, 37.37851562608393863, -13.14518615778179544 ) ) ;
#11407=DIRECTION ( 'NONE',  ( 0.000000000000000000, 1.000000000000000000, 0.000000000000000000 ) ) ;
#11414=EDGE_CURVE ( 'NONE', #8614, #10542, #7856, .T. ) ;
#11417=CARTESIAN_POINT ( 'NONE',  ( 9.295050272127047819, 35.29492187608393294, 9.295050272127046043 ) ) ;
#11420=LINE ( 'NONE', #7010, #7988 ) ;
#11445=CARTESIAN_POINT ( 'NONE',  ( 2.816687638038913930E-15, 20.53589838486225361, -23.00000000000001421 ) ) ;
#11460=ORIENTED_EDGE ( 'NONE', *, *, #7622, .F. ) ;
#11464=CARTESIAN_POINT ( 'NONE',  ( -13.14518615778179189, 36.63437500108393152, 5.444914386472304635 ) ) ;
#11468=FACE_OUTER_BOUND ( 'NONE', #17812, .T. ) ;
#11487=CARTESIAN_POINT ( 'NONE',  ( 9.598844408820456309, 38.42031250216787441, -9.598844408820458085 ) ) ;
#11494=DIRECTION ( 'NONE',  ( 0.000000000000000000, 0.000000000000000000, -1.000000000000000000 ) ) ;
#11496=CARTESIAN_POINT ( 'NONE',  ( 9.598844408820459861, 34.15390624999999858, 9.598844408820456309 ) ) ;
#11498=CARTESIAN_POINT ( 'NONE',  ( 13.14518615778179900, 34.84843750108393579, -5.444914386472297529 ) ) ;
#11501=CARTESIAN_POINT ( 'NONE',  ( 5.622872871577878406, 34.99726562716787726, 13.57481594606304576 ) ) ;
#11520=CARTESIAN_POINT ( 'NONE',  ( 9.598844408820459861, 32.66562500216787157, 9.598844408820456309 ) ) ;
#11523=CARTESIAN_POINT ( 'NONE',  ( -5.444914386472297529, 35.84062500108394289, -13.14518615778179900 ) ) ;
#11527=FACE_OUTER_BOUND ( 'NONE', #20209, .T. ) ;
#11528=CARTESIAN_POINT ( 'NONE',  ( -8.312177448680279460E-16, 34.45156249999999432, -13.57481594606304576 ) ) ;
#11532=( BOUNDED_CURVE ( )  B_SPLINE_CURVE ( 2, ( #13809, #24375, #13378, #15381, #2999, #4864, #6979, #13232, #2859 ),
 .UNSPECIFIED., .F., .F. ) 
 B_SPLINE_CURVE_WITH_KNOTS ( ( 3, 2, 2, 2, 3 ),
 ( 0.8958333333333335924, 0.9062500000000002220, 0.9166666666666667407, 0.9270833333333334814, 0.9375000000000000000 ),
 .UNSPECIFIED. ) 
 CURVE ( )  GEOMETRIC_REPRESENTATION_ITEM ( )  RATIONAL_B_SPLINE_CURVE ( ( 0.9999999999999983347, 0.9238795325112884038, 1.000000000000000000, 0.9238795325112867385, 1.000000000000000000, 0.9238795325112867385, 1.000000000000000000, 0.9238795325112867385, 1.000000000000000000 ) ) 
 REPRESENTATION_ITEM ( '' )  );
#11554=VERTEX_POINT ( 'NONE', #19886 ) ;
#11556=CARTESIAN_POINT ( 'NONE',  ( -5.444914386472299306, 35.14609375108393152, 13.14518615778179722 ) ) ;
#11602=CARTESIAN_POINT ( 'NONE',  ( -13.14518615778179900, 36.53515625108392584, -5.444914386472297529 ) ) ;
#11603=CARTESIAN_POINT ( 'NONE',  ( 0.000000000000000000, 36.00000000000000000, -13.57481594606304576 ) ) ;
#11625=CARTESIAN_POINT ( 'NONE',  ( -9.295050272127044266, 32.11992187608393579, 9.295050272127047819 ) ) ;
#11628=DIRECTION ( 'NONE',  ( 0.000000000000000000, 1.000000000000000000, 0.000000000000000000 ) ) ;
#11637=CARTESIAN_POINT ( 'NONE',  ( 13.57481594606304576, 32.66562499999999858, -1.662435489736055892E-15 ) ) ;
#11639=CARTESIAN_POINT ( 'NONE',  ( -5.444914386472297529, 35.84062500108394289, -13.14518615778179900 ) ) ;
#11641=CARTESIAN_POINT ( 'NONE',  ( 13.14518615778179722, 35.34453125108392157, 5.444914386472293977 ) ) ;
#11642=CARTESIAN_POINT ( 'NONE',  ( 13.57481594606304931, 36.68398437716788152, 5.622872871577869525 ) ) ;
#11668=CARTESIAN_POINT ( 'NONE',  ( -9.295050272127046043, 35.09648437608393579, -9.295050272127046043 ) ) ;
#11689=DIRECTION ( 'NONE',  ( 0.000000000000000000, 0.000000000000000000, 1.000000000000000000 ) ) ;
#11693=LINE ( 'NONE', #1319, #17633 ) ;
#11697=CARTESIAN_POINT ( 'NONE',  ( 2.414731522848535132E-15, 35.98945312608393010, 13.14518615778179544 ) ) ;
#11748=EDGE_CURVE ( 'NONE', #10079, #1506, #20601, .T. ) ;
#11760=ORIENTED_EDGE ( 'NONE', *, *, #14543, .T. ) ;
#11769=CARTESIAN_POINT ( 'NONE',  ( -13.14518615778179189, 32.07031250108393294, 5.444914386472304635 ) ) ;
#11772=CARTESIAN_POINT ( 'NONE',  ( 9.598844408820456309, 40.00781250216787299, -9.598844408820458085 ) ) ;
#11773=AXIS2_PLACEMENT_3D ( 'NONE', #8667, #2122, #19639 ) ;
#11776=CARTESIAN_POINT ( 'NONE',  ( -13.57481594606304398, 33.21132812716787441, 5.622872871577880183 ) ) ;
#11780=CARTESIAN_POINT ( 'NONE',  ( -13.57481594606304576, 35.44374999999999432, 0.000000000000000000 ) ) ;
#11782=CARTESIAN_POINT ( 'NONE',  ( 9.598844408820456309, 33.55859375000000000, -9.598844408820458085 ) ) ;
#11784=CARTESIAN_POINT ( 'NONE',  ( -9.295050272127044266, 35.29492187608393294, 9.295050272127047819 ) ) ;
#11786=CARTESIAN_POINT ( 'NONE',  ( 2.414731522848535132E-15, 35.19570312608392726, 13.14518615778179544 ) ) ;
#11788=CARTESIAN_POINT ( 'NONE',  ( -9.598844408820458085, 37.03125000216787299, -9.598844408820458085 ) ) ;
#11809=VERTEX_POINT ( 'NONE', #25567 ) ;
#11814=CARTESIAN_POINT ( 'NONE',  ( -5.444914386472297529, 36.63437500108393152, -13.14518615778179900 ) ) ;
#11834=CARTESIAN_POINT ( 'NONE',  ( 0.000000000000000000, 11.00000000000000355, 0.000000000000000000 ) ) ;
#11836=DIRECTION ( 'NONE',  ( -0.000000000000000000, -1.000000000000000000, -0.000000000000000000 ) ) ;
#11845=CARTESIAN_POINT ( 'NONE',  ( -13.14518615778179544, 37.37851562608393863, 0.000000000000000000 ) ) ;
#11890=ADVANCED_FACE ( 'NONE', ( #5496 ), #14716, .T. ) ;
#11904=EDGE_CURVE ( 'NONE', #26666, #8864, #17324, .T. ) ;
#11914=CARTESIAN_POINT ( 'NONE',  ( -13.57481594606304576, 37.97382812716787726, 5.622872871577880183 ) ) ;
#11923=CARTESIAN_POINT ( 'NONE',  ( -9.598844408820454532, 35.54296874999999289, 9.598844408820459861 ) ) ;
#11925=CARTESIAN_POINT ( 'NONE',  ( 5.444914386472297529, 34.94765625108394147, -13.14518615778179900 ) ) ;
#11927=CARTESIAN_POINT ( 'NONE',  ( -13.14518615778179722, 34.15390625108393863, -5.444914386472297529 ) ) ;
#11928=CARTESIAN_POINT ( 'NONE',  ( -8.312177448680279460E-16, 35.34453125216787583, -13.57481594606304576 ) ) ;
#11933=DIRECTION ( 'NONE',  ( 0.000000000000000000, 1.000000000000000000, 0.000000000000000000 ) ) ;
#11940=EDGE_LOOP ( 'NONE', ( #23039, #4612, #9169, #13434 ) ) ;
#11954=CARTESIAN_POINT ( 'NONE',  ( -13.14518615778179544, 33.60820312608393579, 0.000000000000000000 ) ) ;
#11981=DIRECTION ( 'NONE',  ( -0.000000000000000000, -1.000000000000000000, -0.000000000000000000 ) ) ;
#11985=CARTESIAN_POINT ( 'NONE',  ( 2.414731522848535132E-15, 36.78320312608393294, 13.14518615778179544 ) ) ;
#12004=CARTESIAN_POINT ( 'NONE',  ( 13.57481594606304576, 31.97109375216787441, -1.662435489736055892E-15 ) ) ;
#12007=CARTESIAN_POINT ( 'NONE',  ( 2.493653234604083739E-15, 33.26093749999999716, 13.57481594606304576 ) ) ;
#12015=VECTOR ( 'NONE', #1869, 1000.000000000000000 ) ;
#12020=DIRECTION ( 'NONE',  ( 0.000000000000000000, 0.000000000000000000, -1.000000000000000000 ) ) ;
#12030=CARTESIAN_POINT ( 'NONE',  ( 9.295050272127047819, 40.25585937608393294, 9.295050272127046043 ) ) ;
#12035=ORIENTED_EDGE ( 'NONE', *, *, #18883, .F. ) ;
#12044=CARTESIAN_POINT ( 'NONE',  ( -13.14518615778179544, 32.02070312608393010, 0.000000000000000000 ) ) ;
#12047=VERTEX_POINT ( 'NONE', #6318 ) ;
#12048=CARTESIAN_POINT ( 'NONE',  ( -9.598844408820458085, 33.75703124999999005, -9.598844408820458085 ) ) ;
#12056=CARTESIAN_POINT ( 'NONE',  ( 5.622872871577878406, 33.31054687499999289, 13.57481594606304576 ) ) ;
#12059=CARTESIAN_POINT ( 'NONE',  ( -13.09590655363597733, 36.00000000000000000, 1.137167824541468031 ) ) ;
#12060=CARTESIAN_POINT ( 'NONE',  ( 5.622872871577878406, 40.45429687500001137, 13.57481594606304576 ) ) ;
#12063=CARTESIAN_POINT ( 'NONE',  ( 13.57481594606304576, 34.35234375216787583, -1.662435489736055892E-15 ) ) ;
#12069=CARTESIAN_POINT ( 'NONE',  ( 13.57481594606304576, 35.14609375216787157, -1.662435489736055892E-15 ) ) ;
#12076=AXIS2_PLACEMENT_3D ( 'NONE', #6436, #12827, #11114 ) ;
#12087=CARTESIAN_POINT ( 'NONE',  ( -5.444914386472299306, 32.96328125108393436, 13.14518615778179722 ) ) ;
#12091=CARTESIAN_POINT ( 'NONE',  ( 2.493653234604083739E-15, 35.74140625216787015, 13.57481594606304576 ) ) ;
#12113=( BOUNDED_CURVE ( )  B_SPLINE_CURVE ( 2, ( #21402, #21534, #23673, #17243, #10543, #26230, #3867, #8838, #2299, #19669, #17098, #4151, #10679, #16962, #19110, #13084, #10815, #19250, #17528, #8409, #6420, #23394, #12811, #23950, #6278, #23808, #6144, #12529, #25801, #25661, #27818, #8554, #15089, #21823, #12943, #21678, #2153, #19530, #23534, #8696, #14809, #26085, #12, #6552, #4432, #6834, #16198, #25043, #3243, #20494, #7358, #13228, #9784, #2439, #3103, #3374, #18493, #14054, #5526, #20633, #26913, #9644, #13373, #19812, #13906, #15524, #24761, #21960, #16051, #18631, #11100, #24232, #14193, #15377, #17669, #1116, #9915, #977, #22912, #22634, #11625, #11769, #12044, #20769, #20349, #27053, #4713, #18348, #7504 ),
 .UNSPECIFIED., .F., .T. ) 
 B_SPLINE_CURVE_WITH_KNOTS ( ( 3, 2, 2, 2, 2, 2, 2, 2, 2, 2, 2, 2, 2, 2, 2, 2, 2, 2, 2, 2, 2, 2, 2, 2, 2, 2, 2, 2, 2, 2, 2, 2, 2, 2, 2, 2, 2, 2, 2, 2, 2, 2, 2, 2, 3 ),
 ( 0.4988304892921909817, 0.5000000000000000000, 0.5104166666666666297, 0.5208333333333333703, 0.5312500000000000000, 0.5416666666666666297, 0.5520833333333333703, 0.5625000000000000000, 0.5729166666666666297, 0.5833333333333333703, 0.5937500000000000000, 0.6041666666666666297, 0.6145833333333333703, 0.6250000000000000000, 0.6354166666666666297, 0.6458333333333333703, 0.6562500000000000000, 0.6666666666666666297, 0.6770833333333333703, 0.6875000000000000000, 0.6979166666666666297, 0.7083333333333333703, 0.7187500000000000000, 0.7291666666666666297, 0.7395833333333333703, 0.7500000000000000000, 0.7604166666666666297, 0.7708333333333333703, 0.7812500000000000000, 0.7916666666666666297, 0.8020833333333333703, 0.8125000000000000000, 0.8229166666666666297, 0.8333333333333333703, 0.8437500000000000000, 0.8541666666666666297, 0.8645833333333334814, 0.8750000000000000000, 0.8854166666666666297, 0.8958333333333333703, 0.9062500000000000000, 0.9166666666666666297, 0.9270833333333333703, 0.9375000000000000000, 0.9448587001587775980 ),
 .UNSPECIFIED. ) 
 CURVE ( )  GEOMETRIC_REPRESENTATION_ITEM ( )  RATIONAL_B_SPLINE_CURVE ( ( 0.9848264816800353927, 0.9914537246260980430, 1.000000000000000000, 0.9238795325112867385, 1.000000000000000000, 0.9238795325112867385, 1.000000000000000000, 0.9238795325112867385, 1.000000000000000000, 0.9238795325112867385, 1.000000000000000000, 0.9238795325112867385, 1.000000000000000000, 0.9238795325112867385, 1.000000000000000000, 0.9238795325112867385, 1.000000000000000000, 0.9238795325112867385, 1.000000000000000000, 0.9238795325112867385, 1.000000000000000000, 0.9238795325112867385, 1.000000000000000000, 0.9238795325112867385, 1.000000000000000000, 0.9238795325112867385, 1.000000000000000000, 0.9238795325112867385, 1.000000000000000000, 0.9238795325112867385, 1.000000000000000000, 0.9238795325112867385, 1.000000000000000000, 0.9238795325112867385, 1.000000000000000000, 0.9238795325112867385, 1.000000000000000000, 0.9238795325112867385, 1.000000000000000000, 0.9238795325112867385, 1.000000000000000000, 0.9238795325112867385, 1.000000000000000000, 0.9238795325112867385, 1.000000000000000000, 0.9238795325112867385, 1.000000000000000000, 0.9238795325112867385, 1.000000000000000000, 0.9238795325112867385, 1.000000000000000000, 0.9238795325112867385, 1.000000000000000000, 0.9238795325112867385, 1.000000000000000000, 0.9238795325112867385, 1.000000000000000000, 0.9238795325112867385, 1.000000000000000000, 0.9238795325112867385, 1.000000000000000000, 0.9238795325112867385, 1.000000000000000000, 0.9238795325112867385, 1.000000000000000000, 0.9238795325112867385, 1.000000000000000000, 0.9238795325112867385, 1.000000000000000000, 0.9238795325112867385, 1.000000000000000000, 0.9238795325112867385, 1.000000000000000000, 0.9238795325112867385, 1.000000000000000000, 0.9238795325112867385, 1.000000000000000000, 0.9238795325112867385, 1.000000000000000000, 0.9238795325112867385, 1.000000000000000000, 0.9238795325112867385, 1.000000000000000000, 0.9238795325112867385, 1.000000000000000000, 0.9238795325112867385, 1.000000000000000000, 0.9462258211652395667, 0.9684275895297407288 ) ) 
 REPRESENTATION_ITEM ( '' )  );
#12114=VERTEX_POINT ( 'NONE', #12849 ) ;
#12119=CARTESIAN_POINT ( 'NONE',  ( 13.14518615778179900, 34.65000000108393152, -5.444914386472297529 ) ) ;
#12126=CARTESIAN_POINT ( 'NONE',  ( 0.000000000000000000, 23.00000000000000000, 0.000000000000000000 ) ) ;
#12132=CARTESIAN_POINT ( 'NONE',  ( -9.295050272127044266, 35.09648437608392868, 9.295050272127047819 ) ) ;
#12134=EDGE_CURVE ( 'NONE', #22508, #8637, #23674, .T. ) ;
#12136=VERTEX_POINT ( 'NONE', #19710 ) ;
#12144=EDGE_LOOP ( 'NONE', ( #20535, #25849, #4452, #26601 ) ) ;
#12148=B_SPLINE_CURVE_WITH_KNOTS ( 'NONE', 3,
 ( #23770, #11059, #12906, #400, #19631, #13336, #19770, #253, #10922, #8937, #4818, #19916, #22063, #17627, #22201, #17204, #13478, #6794, #8658, #23909, #15481, #17349, #4674, #21639, #2540, #10644, #26045, #13046, #19350, #28052, #21781 ),
 .UNSPECIFIED., .F., .F.,
 ( 4, 2, 2, 2, 2, 2, 2, 2, 2, 2, 1, 2, 2, 2, 2, 4 ),
 ( 1.033534235789917861E-15, 0.001647793485001597738, 0.003295586970002162015, 0.004943380455002727158, 0.005767277197503011682, 0.006591173940003295338, 0.008238967425003861783, 0.009886760910004429095, 0.01318234788000556545, 0.01483014136500612756, 0.01647793485000669314, 0.01812572833500725872, 0.01977352182000782083, 0.02306910879000895198, 0.02471690227500952103, 0.02636469576001009008 ),
 .UNSPECIFIED. ) ;
#12165=CARTESIAN_POINT ( 'NONE',  ( -8.049105076161786076E-16, 39.75976562608394005, -13.14518615778179544 ) ) ;
#12193=CARTESIAN_POINT ( 'NONE',  ( -5.622872871577873077, 32.41757812499999858, 13.57481594606304753 ) ) ;
#12195=CARTESIAN_POINT ( 'NONE',  ( -11.93524237669063126, 36.00000000000001421, -5.809862729998008568 ) ) ;
#12197=CARTESIAN_POINT ( 'NONE',  ( -9.598844408820458085, 39.31328124999999574, -9.598844408820458085 ) ) ;
#12198=CARTESIAN_POINT ( 'NONE',  ( 3.755638265659908104, 31.58960998161716560, -13.14518615778179722 ) ) ;
#12199=CARTESIAN_POINT ( 'NONE',  ( 9.598844408820456309, 34.45156250216787441, -9.598844408820458085 ) ) ;
#12204=CARTESIAN_POINT ( 'NONE',  ( 9.598844408820459861, 35.04687500216787299, 9.598844408820456309 ) ) ;
#12222=CARTESIAN_POINT ( 'NONE',  ( 9.295050272127047819, 34.69960937608393436, 9.295050272127046043 ) ) ;
#12224=CARTESIAN_POINT ( 'NONE',  ( 13.57481594606304576, 35.96878166419460143, -3.279908293447338696 ) ) ;
#12256=CARTESIAN_POINT ( 'NONE',  ( 2.414731522848535132E-15, 33.60820312608392868, 13.14518615778179544 ) ) ;
#12271=CARTESIAN_POINT ( 'NONE',  ( 9.295050272127046043, 37.08085937608393579, -9.295050272127046043 ) ) ;
#12272=CARTESIAN_POINT ( 'NONE',  ( 6.944423797152706079, 31.55306878032414986, -11.16113333171310451 ) ) ;
#12305=CARTESIAN_POINT ( 'NONE',  ( -8.312177448680279460E-16, 33.75703125216787726, -13.57481594606304576 ) ) ;
#12308=CARTESIAN_POINT ( 'NONE',  ( 13.14518615778179544, 40.35507812608393863, -1.609821015232357215E-15 ) ) ;
#12329=EDGE_CURVE ( 'NONE', #18468, #12537, #27138, .T. ) ;
#12343=CARTESIAN_POINT ( 'NONE',  ( 13.57481594606304931, 39.75976562499999289, 5.622872871577869525 ) ) ;
#12344=CARTESIAN_POINT ( 'NONE',  ( 9.295050272127046043, 33.90585937608393152, -9.295050272127046043 ) ) ;
#12345=CARTESIAN_POINT ( 'NONE',  ( -5.622872871577873077, 33.01289062716787726, -13.57481594606304753 ) ) ;
#12350=CARTESIAN_POINT ( 'NONE',  ( 9.598844408820456309, 35.24531250216787726, -9.598844408820458085 ) ) ;
#12366=CARTESIAN_POINT ( 'NONE',  ( -5.444914386472297529, 33.45937500108394147, -13.14518615778179900 ) ) ;
#12373=DIRECTION ( 'NONE',  ( -0.000000000000000000, -1.000000000000000000, -0.000000000000000000 ) ) ;
#12380=EDGE_CURVE ( 'NONE', #4040, #19447, #21450, .T. ) ;
#12388=CARTESIAN_POINT ( 'NONE',  ( 3.061616997868384226E-15, 23.00000000000000000, 25.00000000000001066 ) ) ;
#12395=CARTESIAN_POINT ( 'NONE',  ( 2.414731522848535132E-15, 34.40195312608393152, 13.14518615778179544 ) ) ;
#12404=AXIS2_PLACEMENT_3D ( 'NONE', #2184, #26262, #15118 ) ;
#12412=CARTESIAN_POINT ( 'NONE',  ( 5.444914386472297529, 33.95546875108393436, -13.14518615778179900 ) ) ;
#12458=CARTESIAN_POINT ( 'NONE',  ( 0.000000000000000000, 21.95886589889650509, -23.00000000000001421 ) ) ;
#12470=ORIENTED_EDGE ( 'NONE', *, *, #22061, .T. ) ;
#12472=CARTESIAN_POINT ( 'NONE',  ( -9.295050272127046043, 32.71523437608393436, -9.295050272127046043 ) ) ;
#12473=CARTESIAN_POINT ( 'NONE',  ( 13.14518615778179722, 33.85625000108393579, -5.444914386472297529 ) ) ;
#12474=CARTESIAN_POINT ( 'NONE',  ( 9.598844408820456309, 32.86406250216787583, -9.598844408820458085 ) ) ;
#12485=ORIENTED_EDGE ( 'NONE', *, *, #16095, .T. ) ;
#12520=DIRECTION ( 'NONE',  ( 0.000000000000000000, 1.000000000000000000, 0.000000000000000000 ) ) ;
#12529=CARTESIAN_POINT ( 'NONE',  ( 13.14518615778179722, 34.74921875108395142, 5.444914386472293977 ) ) ;
#12530=CARTESIAN_POINT ( 'NONE',  ( 13.14518615778179900, 32.96328125108393436, 5.444914386472293977 ) ) ;
#12537=VERTEX_POINT ( 'NONE', #4020 ) ;
#12539=TOROIDAL_SURFACE ( 'NONE', #743, 23.26794919243112858, 1.000000000000000000 ) ;
#12546=CARTESIAN_POINT ( 'NONE',  ( -13.14518615778179544, 31.82226562608393650, 0.000000000000000000 ) ) ;
#12557=AXIS2_PLACEMENT_3D ( 'NONE', #7535, #16372, #20664 ) ;
#12599=EDGE_CURVE ( 'NONE', #5426, #18529, #10826, .T. ) ;
#12613=CARTESIAN_POINT ( 'NONE',  ( -8.312177448680279460E-16, 40.00781250000000000, -13.57481594606304576 ) ) ;
#12615=CARTESIAN_POINT ( 'NONE',  ( -8.049105076161786076E-16, 31.62382812608393579, -13.14518615778179544 ) ) ;
#12617=CARTESIAN_POINT ( 'NONE',  ( 5.622872871577878406, 31.82226562716787654, 13.57481594606304576 ) ) ;
#12664=AXIS2_PLACEMENT_3D ( 'NONE', #22241, #6831, #580 ) ;
#12668=CARTESIAN_POINT ( 'NONE',  ( -9.598844408820454532, 31.67343750216787512, 9.598844408820459861 ) ) ;
#12677=CARTESIAN_POINT ( 'NONE',  ( 13.14518615778179900, 33.06250000108393294, -5.444914386472297529 ) ) ;
#12693=CARTESIAN_POINT ( 'NONE',  ( 0.000000000000000000, 10.00000000000000178, 16.91709623134523000 ) ) ;
#12704=ORIENTED_EDGE ( 'NONE', *, *, #3565, .T. ) ;
#12707=DIRECTION ( 'NONE',  ( 0.000000000000000000, 0.000000000000000000, 1.000000000000000000 ) ) ;
#12744=VECTOR ( 'NONE', #19397, 1000.000000000000000 ) ;
#12753=ORIENTED_EDGE ( 'NONE', *, *, #18211, .F. ) ;
#12756=CARTESIAN_POINT ( 'NONE',  ( -8.049105076161786076E-16, 34.00507812608393721, -13.14518615778179544 ) ) ;
#12757=CARTESIAN_POINT ( 'NONE',  ( -13.14518615778179544, 40.55351562608393579, 0.000000000000000000 ) ) ;
#12774=ADVANCED_FACE ( 'NONE', ( #9408 ), #3004, .T. ) ;
#12789=CARTESIAN_POINT ( 'NONE',  ( -5.444914386472297529, 37.42812500108394147, -13.14518615778179900 ) ) ;
#12800=ORIENTED_EDGE ( 'NONE', *, *, #19932, .F. ) ;
#12802=DIRECTION ( 'NONE',  ( 0.000000000000000000, 0.000000000000000000, 1.000000000000000000 ) ) ;
#12811=CARTESIAN_POINT ( 'NONE',  ( -8.049105076161786076E-16, 34.99726562608393721, -13.14518615778179544 ) ) ;
#12812=CARTESIAN_POINT ( 'NONE',  ( -13.14518615778179544, 31.82226562608393650, 0.000000000000000000 ) ) ;
#12827=DIRECTION ( 'NONE',  ( -0.000000000000000000, -1.000000000000000000, -0.000000000000000000 ) ) ;
#12829=CARTESIAN_POINT ( 'NONE',  ( -9.295050272127046043, 32.51679687608393721, -9.295050272127046043 ) ) ;
#12849=CARTESIAN_POINT ( 'NONE',  ( -8.312177448680279460E-16, 31.37578125216787583, -13.57481594606304576 ) ) ;
#12851=ORIENTED_EDGE ( 'NONE', *, *, #21718, .T. ) ;
#12859=FACE_OUTER_BOUND ( 'NONE', #15041, .T. ) ;
#12874=CARTESIAN_POINT ( 'NONE',  ( 9.295050272127046043, 33.31054687608394005, -9.295050272127046043 ) ) ;
#12876=EDGE_CURVE ( 'NONE', #6997, #17432, #26422, .T. ) ;
#12888=CARTESIAN_POINT ( 'NONE',  ( 13.14518615778179544, 39.36289062608393152, -1.609821015232357215E-15 ) ) ;
#12906=CARTESIAN_POINT ( 'NONE',  ( 2.232327155338130975, 36.00000000000002132, 12.98409812936875696 ) ) ;
#12917=CARTESIAN_POINT ( 'NONE',  ( -9.598844408820454532, 32.46718750216787441, 9.598844408820459861 ) ) ;
#12918=CARTESIAN_POINT ( 'NONE',  ( -9.598844408820458085, 38.51953124999999289, -9.598844408820458085 ) ) ;
#12920=CARTESIAN_POINT ( 'NONE',  ( 13.14518615778179900, 38.71796875108393721, 5.444914386472293977 ) ) ;
#12936=ORIENTED_EDGE ( 'NONE', *, *, #20813, .T. ) ;
#12943=CARTESIAN_POINT ( 'NONE',  ( -13.14518615778179544, 34.40195312608393152, 0.000000000000000000 ) ) ;
#12944=CARTESIAN_POINT ( 'NONE',  ( -9.295050272127046043, 40.65273437608393436, -9.295050272127046043 ) ) ;
#12949=CARTESIAN_POINT ( 'NONE',  ( 7.171390501253594785, 31.30502191632583830, -11.52591802191987114 ) ) ;
#12956=CARTESIAN_POINT ( 'NONE',  ( 0.000000000000000000, 0.000000000000000000, 25.00000000000000711 ) ) ;
#12965=CARTESIAN_POINT ( 'NONE',  ( 13.14518615778179544, 33.01289062608393010, -1.609821015232357215E-15 ) ) ;
#12974=EDGE_LOOP ( 'NONE', ( #17836, #22942, #15345, #14256 ) ) ;
#12980=CARTESIAN_POINT ( 'NONE',  ( -9.295050272127044266, 38.27148437608393294, 9.295050272127047819 ) ) ;
#12996=VECTOR ( 'NONE', #1148, 1000.000000000000000 ) ;
#13000=ORIENTED_EDGE ( 'NONE', *, *, #5180, .T. ) ;
#13016=CIRCLE ( 'NONE', #25351, 25.00000000000000711 ) ;
#13019=AXIS2_PLACEMENT_3D ( 'NONE', #7630, #16322, #25023 ) ;
#13023=VERTEX_POINT ( 'NONE', #11113 ) ;
#13027=CARTESIAN_POINT ( 'NONE',  ( -9.295050272127046043, 38.86679687608393863, -9.295050272127046043 ) ) ;
#13046=CARTESIAN_POINT ( 'NONE',  ( 12.89215161363535778, 36.00000000000001421, -4.169510824908217117 ) ) ;
#13051=CIRCLE ( 'NONE', #26754, 23.00000000000001421 ) ;
#13056=CARTESIAN_POINT ( 'NONE',  ( -13.57481594606304753, 36.98164062499999005, -5.622872871577873077 ) ) ;
#13058=CARTESIAN_POINT ( 'NONE',  ( 13.14518615778179900, 38.81718750108393579, -5.444914386472297529 ) ) ;
#13084=CARTESIAN_POINT ( 'NONE',  ( -5.444914386472299306, 35.34453125108393579, 13.14518615778179722 ) ) ;
#13085=CARTESIAN_POINT ( 'NONE',  ( -5.444914386472297529, 39.80937500108392868, -13.14518615778179900 ) ) ;
#13120=CARTESIAN_POINT ( 'NONE',  ( -13.14518615778179544, 39.75976562608393294, 0.000000000000000000 ) ) ;
#13121=AXIS2_PLACEMENT_3D ( 'NONE', #10232, #1297, #6117 ) ;
#13129=CARTESIAN_POINT ( 'NONE',  ( -13.57481594606304398, 34.79882812716788010, 5.622872871577880183 ) ) ;
#13163=( LENGTH_UNIT ( ) NAMED_UNIT ( * ) SI_UNIT ( .MILLI., .METRE. ) );
#13169=CARTESIAN_POINT ( 'NONE',  ( -13.14518615778179189, 38.22187500108393010, 5.444914386472304635 ) ) ;
#13192=DIRECTION ( 'NONE',  ( 0.000000000000000000, 1.000000000000000000, 0.000000000000000000 ) ) ;
#13202=CARTESIAN_POINT ( 'NONE',  ( -13.57481594606304576, 37.87460937499999147, 5.622872871577880183 ) ) ;
#13204=CARTESIAN_POINT ( 'NONE',  ( 2.414731522848535132E-15, 36.98164062608393721, 13.14518615778179544 ) ) ;
#13225=CARTESIAN_POINT ( 'NONE',  ( 13.57481594606304931, 32.71523437716787441, 5.622872871577868636 ) ) ;
#13228=CARTESIAN_POINT ( 'NONE',  ( -13.14518615778179722, 33.55859375108393294, -5.444914386472297529 ) ) ;
#13229=CARTESIAN_POINT ( 'NONE',  ( -13.14518615778179189, 39.21406250108392300, 5.444914386472304635 ) ) ;
#13232=CARTESIAN_POINT ( 'NONE',  ( -5.622872871577873966, 32.11992187499999574, -13.57481594606304753 ) ) ;
#13249=ORIENTED_EDGE ( 'NONE', *, *, #22715, .T. ) ;
#13260=CARTESIAN_POINT ( 'NONE',  ( 13.14518615778179900, 38.61875000108393152, -5.444914386472297529 ) ) ;
#13284=EDGE_CURVE ( 'NONE', #12047, #22508, #36, .T. ) ;
#13301=CARTESIAN_POINT ( 'NONE',  ( 0.000000000000000000, 1.500000000000001332, 0.000000000000000000 ) ) ;
#13314=AXIS2_PLACEMENT_3D ( 'NONE', #5222, #26608, #16177 ) ;
#13315=CARTESIAN_POINT ( 'NONE',  ( 9.295050272127047819, 37.67617187608393436, 9.295050272127046043 ) ) ;
#13336=CARTESIAN_POINT ( 'NONE',  ( 4.859977269582195447, 36.00000000000000000, 12.29462155906275100 ) ) ;
#13345=CARTESIAN_POINT ( 'NONE',  ( -13.57481594606304398, 32.41757812716787868, 5.622872871577880183 ) ) ;
#13346=CARTESIAN_POINT ( 'NONE',  ( 13.57481594606304576, 38.22187499999999716, -1.662435489736055892E-15 ) ) ;
#13348=CARTESIAN_POINT ( 'NONE',  ( -9.295050272127046043, 37.47773437608393010, -9.295050272127046043 ) ) ;
#13370=DIRECTION ( 'NONE',  ( 1.000000000000000000, -0.000000000000000000, 1.224646799147353207E-16 ) ) ;
#13373=CARTESIAN_POINT ( 'NONE',  ( 2.414731522848535132E-15, 33.01289062608393721, 13.14518615778179544 ) ) ;
#13374=CARTESIAN_POINT ( 'NONE',  ( 5.444914386472302859, 38.61875000108393152, 13.14518615778179189 ) ) ;
#13376=VERTEX_POINT ( 'NONE', #22655 ) ;
#13378=CARTESIAN_POINT ( 'NONE',  ( -9.598844408820454532, 32.36796874999999574, 9.598844408820459861 ) ) ;
#13404=EDGE_LOOP ( 'NONE', ( #8649, #10225, #12704, #16841 ) ) ;
#13407=CARTESIAN_POINT ( 'NONE',  ( 5.444914386472297529, 40.30546875108393579, -13.14518615778179900 ) ) ;
#13434=ORIENTED_EDGE ( 'NONE', *, *, #9151, .F. ) ;
#13450=AXIS2_PLACEMENT_3D ( 'NONE', #19757, #17615, #26323 ) ;
#13455=CARTESIAN_POINT ( 'NONE',  ( 9.295050272127047819, 34.50117187608393010, 9.295050272127046043 ) ) ;
#13467=ORIENTED_EDGE ( 'NONE', *, *, #11748, .T. ) ;
#13468=CARTESIAN_POINT ( 'NONE',  ( 9.598844408820456309, 33.55859375000000000, -9.598844408820458085 ) ) ;
#13474=ADVANCED_FACE ( 'NONE', ( #22797 ), #1841, .T. ) ;
#13478=CARTESIAN_POINT ( 'NONE',  ( 11.20653150213565041, 36.00000000000000711, 7.323573988460845285 ) ) ;
#13480=CONICAL_SURFACE ( 'NONE', #15771, 17.49444650053485972, 0.5235987755983000369 ) ;
#13483=CARTESIAN_POINT ( 'NONE',  ( 5.622872871577871301, 38.46992187716787015, -13.57481594606304753 ) ) ;
#13491=CARTESIAN_POINT ( 'NONE',  ( 0.000000000000000000, 36.00000000000000000, 0.000000000000000000 ) ) ;
#13493=CARTESIAN_POINT ( 'NONE',  ( -5.622872871577873077, 38.46992187499999716, -13.57481594606304753 ) ) ;
#13496=CARTESIAN_POINT ( 'NONE',  ( 9.295050272127046043, 33.31054687608394005, -9.295050272127046043 ) ) ;
#13499=CARTESIAN_POINT ( 'NONE',  ( -5.622872871577873077, 37.27929687716787299, 13.57481594606304753 ) ) ;
#13510=ORIENTED_EDGE ( 'NONE', *, *, #24310, .T. ) ;
#13512=CARTESIAN_POINT ( 'NONE',  ( -8.312177448680279460E-16, 35.24531249999999716, -13.57481594606304576 ) ) ;
#13525=CARTESIAN_POINT ( 'NONE',  ( -13.14518615778179189, 35.24531250108393721, 5.444914386472304635 ) ) ;
#13547=LINE ( 'NONE', #22270, #252 ) ;
#13555=CARTESIAN_POINT ( 'NONE',  ( 5.444914386472302859, 37.62656250108393863, 13.14518615778179189 ) ) ;
#13587=ORIENTED_EDGE ( 'NONE', *, *, #24186, .T. ) ;
#13604=CARTESIAN_POINT ( 'NONE',  ( 13.14518615778179900, 34.55078125108393294, 5.444914386472293977 ) ) ;
#13628=CARTESIAN_POINT ( 'NONE',  ( -9.598844408820458085, 39.41250000216787441, -9.598844408820458085 ) ) ;
#13636=FACE_OUTER_BOUND ( 'NONE', #14802, .T. ) ;
#13638=CARTESIAN_POINT ( 'NONE',  ( -9.598844408820458085, 34.55078124999999289, -9.598844408820458085 ) ) ;
#13640=CARTESIAN_POINT ( 'NONE',  ( -9.295050272127046043, 35.09648437608393579, -9.295050272127046043 ) ) ;
#13643=CARTESIAN_POINT ( 'NONE',  ( 13.14518615778179722, 34.55078125108393294, 5.444914386472293977 ) ) ;
#13644=CARTESIAN_POINT ( 'NONE',  ( 5.622872871577871301, 36.08867187716787583, -13.57481594606304753 ) ) ;
#13656=CARTESIAN_POINT ( 'NONE',  ( 13.57481594606304576, 35.04687499999999289, -1.662435489736055892E-15 ) ) ;
#13668=CARTESIAN_POINT ( 'NONE',  ( 5.444914386472302859, 36.23750000108393721, 13.14518615778179189 ) ) ;
#13672=EDGE_CURVE ( 'NONE', #8864, #4666, #15479, .T. ) ;
#13677=DIRECTION ( 'NONE',  ( -0.000000000000000000, -1.000000000000000000, -0.000000000000000000 ) ) ;
#13692=TOROIDAL_SURFACE ( 'NONE', #1436, 23.26794919243112503, 1.000000000000000000 ) ;
#13699=CARTESIAN_POINT ( 'NONE',  ( 2.414731522848535132E-15, 35.19570312608392726, 13.14518615778179544 ) ) ;
#13735=CARTESIAN_POINT ( 'NONE',  ( -13.57481594606304576, 33.95546875216787441, 0.000000000000000000 ) ) ;
#13740=CARTESIAN_POINT ( 'NONE',  ( -2.849501950123402991E-15, -1.000000000000001998, -23.26794919243113213 ) ) ;
#13743=CARTESIAN_POINT ( 'NONE',  ( -5.444914386472299306, 35.14609375108393152, 13.14518615778179722 ) ) ;
#13750=CARTESIAN_POINT ( 'NONE',  ( 7.114649318941503431, 31.93754143773660203, -11.43472154218138570 ) ) ;
#13766=CARTESIAN_POINT ( 'NONE',  ( 2.493653234604083739E-15, 38.91640625216786731, 13.57481594606304576 ) ) ;
#13773=DIRECTION ( 'NONE',  ( -0.000000000000000000, -1.000000000000000000, -0.000000000000000000 ) ) ;
#13775=CARTESIAN_POINT ( 'NONE',  ( -8.312177448680279460E-16, 32.86406249999999574, -13.57481594606304576 ) ) ;
#13776=CARTESIAN_POINT ( 'NONE',  ( 6.944423797152706079, 31.55306878032414986, -11.16113333171310451 ) ) ;
#13777=CARTESIAN_POINT ( 'NONE',  ( -8.049105076161786076E-16, 34.99726562608393721, -13.14518615778179544 ) ) ;
#13779=CARTESIAN_POINT ( 'NONE',  ( 2.414731522848535132E-15, 34.40195312608393152, 13.14518615778179544 ) ) ;
#13780=CARTESIAN_POINT ( 'NONE',  ( -13.57481594606304753, 34.69960937716787441, -5.622872871577873077 ) ) ;
#13805=CARTESIAN_POINT ( 'NONE',  ( 5.444914386472297529, 37.32890625108393579, -13.14518615778179900 ) ) ;
#13809=CARTESIAN_POINT ( 'NONE',  ( 2.493653234604083739E-15, 32.46718749999999432, 13.57481594606304576 ) ) ;
#13821=DIRECTION ( 'NONE',  ( 0.000000000000000000, 0.000000000000000000, 1.000000000000000000 ) ) ;
#13836=CARTESIAN_POINT ( 'NONE',  ( -13.14518615778179900, 37.32890625108393579, -5.444914386472297529 ) ) ;
#13884=CARTESIAN_POINT ( 'NONE',  ( -9.598844408820458085, 35.44375000216787441, -9.598844408820458085 ) ) ;
#13891=CIRCLE ( 'NONE', #5731, 11.57481594606304576 ) ;
#13906=CARTESIAN_POINT ( 'NONE',  ( -9.295050272127044266, 32.91367187608393152, 9.295050272127047819 ) ) ;
#13911=CIRCLE ( 'NONE', #3924, 23.00000000000001421 ) ;
#13918=CARTESIAN_POINT ( 'NONE',  ( 13.57481594606304753, 35.09648437499998863, -5.622872871577873077 ) ) ;
#13919=CARTESIAN_POINT ( 'NONE',  ( -9.295050272127046043, 35.89023437608393152, -9.295050272127046043 ) ) ;
#13921=CARTESIAN_POINT ( 'NONE',  ( 13.14518615778179544, 35.39414062608393152, -1.609821015232357215E-15 ) ) ;
#13922=CARTESIAN_POINT ( 'NONE',  ( 13.57481594606304576, 37.52734375216787299, -1.662435489736055892E-15 ) ) ;
#13923=LINE ( 'NONE', #27072, #6728 ) ;
#13947=CARTESIAN_POINT ( 'NONE',  ( -9.295050272127046043, 35.89023437608393152, -9.295050272127046043 ) ) ;
#13949=( BOUNDED_CURVE ( )  B_SPLINE_CURVE ( 2, ( #14945, #23524, #12668, #20975, #18960, #21392, #23115, #16826, #6001 ),
 .UNSPECIFIED., .F., .T. ) 
 B_SPLINE_CURVE_WITH_KNOTS ( ( 3, 2, 2, 2, 3 ),
 ( 0.8958333333333335924, 0.9062500000000002220, 0.9166666666666667407, 0.9270833333333334814, 0.9375000000000000000 ),
 .UNSPECIFIED. ) 
 CURVE ( )  GEOMETRIC_REPRESENTATION_ITEM ( )  RATIONAL_B_SPLINE_CURVE ( ( 0.9999999999999983347, 0.9238795325112884038, 1.000000000000000000, 0.9238795325112867385, 1.000000000000000000, 0.9238795325112867385, 1.000000000000000000, 0.9238795325112867385, 1.000000000000000000 ) ) 
 REPRESENTATION_ITEM ( '' )  );
#13951=DIRECTION ( 'NONE',  ( -0.000000000000000000, -1.000000000000000000, -0.000000000000000000 ) ) ;
#13968=ORIENTED_EDGE ( 'NONE', *, *, #10318, .F. ) ;
#13977=CARTESIAN_POINT ( 'NONE',  ( 9.295050272127046043, 37.87460937608393152, -9.295050272127046043 ) ) ;
#13995=PRODUCT_DEFINITION_SHAPE ( 'NONE', 'NONE',  #9428 ) ;
#13999=ADVANCED_FACE ( 'NONE', ( #12859 ), #15002, .F. ) ;
#14008=EDGE_LOOP ( 'NONE', ( #3479, #3448, #9881, #6459 ) ) ;
#14012=ADVANCED_FACE ( 'NONE', ( #3923 ), #15143, .F. ) ;
#14024=ORIENTED_EDGE ( 'NONE', *, *, #17684, .T. ) ;
#14033=DIRECTION ( 'NONE',  ( 0.000000000000000000, 1.000000000000000000, 0.000000000000000000 ) ) ;
#14054=CARTESIAN_POINT ( 'NONE',  ( 13.14518615778179722, 33.26093750108393721, -5.444914386472297529 ) ) ;
#14057=EDGE_LOOP ( 'NONE', ( #22845, #23586, #12470, #15228 ) ) ;
#14058=CARTESIAN_POINT ( 'NONE',  ( 5.622872871577871301, 40.05742187716786873, -13.57481594606304753 ) ) ;
#14066=CARTESIAN_POINT ( 'NONE',  ( -5.622872871577873077, 34.79882812499998579, 13.57481594606304753 ) ) ;
#14068=CARTESIAN_POINT ( 'NONE',  ( 9.295050272127046043, 34.10429687608393579, -9.295050272127046043 ) ) ;
#14072=CARTESIAN_POINT ( 'NONE',  ( -9.598844408820454532, 35.64218750216787868, 9.598844408820459861 ) ) ;
#14096=CARTESIAN_POINT ( 'NONE',  ( 13.14518615778179900, 36.33671875108394289, 5.444914386472293977 ) ) ;
#14126=CARTESIAN_POINT ( 'NONE',  ( -5.444914386472297529, 38.02343750108394005, -13.14518615778179900 ) ) ;
#14128=CARTESIAN_POINT ( 'NONE',  ( 0.000000000000000000, 20.00000000000000000, 0.000000000000000000 ) ) ;
#14147=CARTESIAN_POINT ( 'NONE',  ( 5.622872871577786924, 31.82226562716788365, 13.57481594606313813 ) ) ;
#14155=CARTESIAN_POINT ( 'NONE',  ( 2.142451790973463043E-15, 11.00000000000000355, -17.49444650053485972 ) ) ;
#14177=CARTESIAN_POINT ( 'NONE',  ( -9.295050272127046043, 40.65273437608393436, -9.295050272127046043 ) ) ;
#14193=CARTESIAN_POINT ( 'NONE',  ( 9.295050272127046043, 32.51679687608393721, -9.295050272127046043 ) ) ;
#14201=FACE_OUTER_BOUND ( 'NONE', #26550, .T. ) ;
#14204=CARTESIAN_POINT ( 'NONE',  ( -5.622872871577873077, 34.00507812499999716, 13.57481594606304753 ) ) ;
#14208=CARTESIAN_POINT ( 'NONE',  ( -9.598844408820458085, 40.10703124999999147, -9.598844408820458085 ) ) ;
#14210=CARTESIAN_POINT ( 'NONE',  ( 13.14518615778179722, 35.44375000108393436, -5.444914386472297529 ) ) ;
#14213=CARTESIAN_POINT ( 'NONE',  ( 9.598844408820459861, 34.25312500216787015, 9.598844408820456309 ) ) ;
#14235=CARTESIAN_POINT ( 'NONE',  ( -9.295050272127046043, 34.30273437608393294, -9.295050272127046043 ) ) ;
#14256=ORIENTED_EDGE ( 'NONE', *, *, #2205, .F. ) ;
#14261=ORIENTED_EDGE ( 'NONE', *, *, #2536, .T. ) ;
#14266=CARTESIAN_POINT ( 'NONE',  ( 13.14518615778179900, 32.16953125108393152, 5.444914386472293977 ) ) ;
#14278=CARTESIAN_POINT ( 'NONE',  ( -5.444914386472297529, 35.64218750108392442, -13.14518615778179900 ) ) ;
#14281=ORIENTED_EDGE ( 'NONE', *, *, #10867, .F. ) ;
#14308=CARTESIAN_POINT ( 'NONE',  ( 0.000000000000000000, 21.36169591142201440, 0.000000000000000000 ) ) ;
#14310=CARTESIAN_POINT ( 'NONE',  ( 5.444914386472297529, 39.71015625108393010, -13.14518615778179900 ) ) ;
#14332=VECTOR ( 'NONE', #3080, 1000.000000000000000 ) ;
#14333=CARTESIAN_POINT ( 'NONE',  ( 2.493653234604083739E-15, 34.05468749999999289, 13.57481594606304576 ) ) ;
#14343=VECTOR ( 'NONE', #4750, 1000.000000000000000 ) ;
#14346=CARTESIAN_POINT ( 'NONE',  ( -13.15267690958718205, 36.00000000000000711, 0.5874252385153145850 ) ) ;
#14347=CARTESIAN_POINT ( 'NONE',  ( -13.57481594606304576, 39.41249999999999432, 0.000000000000000000 ) ) ;
#14348=CARTESIAN_POINT ( 'NONE',  ( -5.444914386472299306, 33.55859375108393294, 13.14518615778179722 ) ) ;
#14349=CARTESIAN_POINT ( 'NONE',  ( -9.598844408820458085, 32.26875000216787726, -9.598844408820458085 ) ) ;
#14374=CARTESIAN_POINT ( 'NONE',  ( -9.295050272127044266, 32.11992187608393579, 9.295050272127047819 ) ) ;
#14397=EDGE_CURVE ( 'NONE', #1506, #18417, #11693, .T. ) ;
#14406=CARTESIAN_POINT ( 'NONE',  ( -5.444914386472299306, 31.97109375108393436, 13.14518615778179722 ) ) ;
#14411=AXIS2_PLACEMENT_3D ( 'NONE', #22754, #9202, #16027 ) ;
#14419=AXIS2_PLACEMENT_3D ( 'NONE', #21837, #23965, #11111 ) ;
#14421=CARTESIAN_POINT ( 'NONE',  ( -5.444914386472299306, 35.93984375108392726, 13.14518615778179722 ) ) ;
#14450=DIRECTION ( 'NONE',  ( 0.000000000000000000, 0.000000000000000000, 1.000000000000000000 ) ) ;
#14453=CARTESIAN_POINT ( 'NONE',  ( -5.444914386472299306, 40.10703125108393152, 13.14518615778179722 ) ) ;
#14458=ORIENTED_EDGE ( 'NONE', *, *, #7410, .F. ) ;
#14459=EDGE_LOOP ( 'NONE', ( #1570, #4473, #22230, #24737 ) ) ;
#14487=CARTESIAN_POINT ( 'NONE',  ( 5.444914386472297529, 32.56640625108394005, -13.14518615778179900 ) ) ;
#14488=CARTESIAN_POINT ( 'NONE',  ( 13.14518615778179722, 33.06250000108393294, -5.444914386472297529 ) ) ;
#14489=CARTESIAN_POINT ( 'NONE',  ( -9.598844408820458085, 33.06250000216787299, -9.598844408820458085 ) ) ;
#14511=CARTESIAN_POINT ( 'NONE',  ( -5.444914386472299306, 33.75703125108393721, 13.14518615778179722 ) ) ;
#14531=VECTOR ( 'NONE', #18331, 1000.000000000000000 ) ;
#14543=EDGE_CURVE ( 'NONE', #20304, #27010, #8423, .T. ) ;
#14546=CARTESIAN_POINT ( 'NONE',  ( -5.444914386472299306, 34.35234375108392868, 13.14518615778179722 ) ) ;
#14555=DIRECTION ( 'NONE',  ( 0.000000000000000000, 0.000000000000000000, 1.000000000000000000 ) ) ;
#14562=CARTESIAN_POINT ( 'NONE',  ( 13.14518615778179544, 33.80664062608393294, -1.609821015232357215E-15 ) ) ;
#14575=ORIENTED_EDGE ( 'NONE', *, *, #21090, .F. ) ;
#14589=CARTESIAN_POINT ( 'NONE',  ( 13.57481594606304931, 34.30273437716787299, 5.622872871577868636 ) ) ;
#14620=CARTESIAN_POINT ( 'NONE',  ( 9.295050272127047819, 32.31835937608393294, 9.295050272127046043 ) ) ;
#14621=CARTESIAN_POINT ( 'NONE',  ( -5.444914386472297529, 34.05468750108393294, -13.14518615778179722 ) ) ;
#14622=CARTESIAN_POINT ( 'NONE',  ( 13.57481594606304753, 34.40195312716787157, -5.622872871577873077 ) ) ;
#14633=CARTESIAN_POINT ( 'NONE',  ( 2.493653234604083739E-15, 33.26093749999999716, 13.57481594606304576 ) ) ;
#14644=CARTESIAN_POINT ( 'NONE',  ( -13.14518615778179189, 32.07031250108393294, 5.444914386472304635 ) ) ;
#14670=CARTESIAN_POINT ( 'NONE',  ( 9.598844408820459861, 32.56640625000000000, 9.598844408820456309 ) ) ;
#14674=CARTESIAN_POINT ( 'NONE',  ( -13.14518615778179900, 34.15390625108393863, -5.444914386472297529 ) ) ;
#14686=EDGE_CURVE ( 'NONE', #19382, #11554, #20890, .T. ) ;
#14691=CARTESIAN_POINT ( 'NONE',  ( -5.444914386472299306, 32.76484375108393010, 13.14518615778179722 ) ) ;
#14700=CARTESIAN_POINT ( 'NONE',  ( 13.57481594606304753, 32.02070312716787015, -5.622872871577873966 ) ) ;
#14704=EDGE_LOOP ( 'NONE', ( #17891, #16556, #4417, #25582 ) ) ;
#14716=CYLINDRICAL_SURFACE ( 'NONE', #5057, 13.57481594606304576 ) ;
#14727=DIRECTION ( 'NONE',  ( -0.000000000000000000, -1.000000000000000000, -0.000000000000000000 ) ) ;
#14737=EDGE_CURVE ( 'NONE', #21429, #8864, #4044, .T. ) ;
#14750=FILL_AREA_STYLE ('',( #11034 ) ) ;
#14755=CARTESIAN_POINT ( 'NONE',  ( -9.598844408820458085, 40.90078124999999432, -9.598844408820458085 ) ) ;
#14756=CARTESIAN_POINT ( 'NONE',  ( -13.14518615778179544, 31.82226562608393650, 0.000000000000000000 ) ) ;
#14757=CARTESIAN_POINT ( 'NONE',  ( 13.57481594606304576, 32.76484375216787015, -1.662435489736055892E-15 ) ) ;
#14780=CARTESIAN_POINT ( 'NONE',  ( 13.57481594606304576, 35.93984375216787441, -1.662435489736055892E-15 ) ) ;
#14801=CARTESIAN_POINT ( 'NONE',  ( 0.000000000000000000, 20.53589838486225361, 0.000000000000000000 ) ) ;
#14802=EDGE_LOOP ( 'NONE', ( #45, #14024, #23997, #7109 ) ) ;
#14809=CARTESIAN_POINT ( 'NONE',  ( 9.295050272127046043, 34.10429687608393579, -9.295050272127046043 ) ) ;
#14810=CARTESIAN_POINT ( 'NONE',  ( -13.14518615778179189, 33.45937500108392726, 5.444914386472304635 ) ) ;
#14818=ADVANCED_FACE ( 'NONE', ( #5001 ), #19453, .T. ) ;
#14828=CARTESIAN_POINT ( 'NONE',  ( -9.295050272127044266, 32.71523437608393436, 9.295050272127047819 ) ) ;
#14844=EDGE_CURVE ( 'NONE', #10542, #27857, #18270, .T. ) ;
#14865=DIRECTION ( 'NONE',  ( -1.003171929053526103E-16, -0.5735764363510443831, -0.8191520442889929088 ) ) ;
#14879=DIRECTION ( 'NONE',  ( 0.000000000000000000, 0.000000000000000000, 1.000000000000000000 ) ) ;
#14894=CARTESIAN_POINT ( 'NONE',  ( 9.295050272127047819, 33.70742187608393436, 9.295050272127046043 ) ) ;
#14896=CARTESIAN_POINT ( 'NONE',  ( 9.295050272127047819, 38.46992187608393010, 9.295050272127046043 ) ) ;
#14929=CARTESIAN_POINT ( 'NONE',  ( -5.444914386472299306, 36.93203125108394147, 13.14518615778179722 ) ) ;
#14937=CARTESIAN_POINT ( 'NONE',  ( -8.125303917791095287, 36.00000000000000000, 10.34220695173585902 ) ) ;
#14941=AXIS2_PLACEMENT_3D ( 'NONE', #1121, #7798, #16486 ) ;
#14945=CARTESIAN_POINT ( 'NONE',  ( 2.493653234604083739E-15, 31.77265625216787370, 13.57481594606304576 ) ) ;
#14953=ORIENTED_EDGE ( 'NONE', *, *, #5353, .F. ) ;
#14955=CARTESIAN_POINT ( 'NONE',  ( 13.14518615778179900, 38.02343750108395426, -5.444914386472297529 ) ) ;
#14973=CARTESIAN_POINT ( 'NONE',  ( -5.444914386472297529, 33.26093750108393721, -13.14518615778179900 ) ) ;
#14984=ORIENTED_EDGE ( 'NONE', *, *, #12380, .F. ) ;
#14990=CARTESIAN_POINT ( 'NONE',  ( 5.444914386472297529, 39.51171875108392584, -13.14518615778179900 ) ) ;
#15002=CONICAL_SURFACE ( 'NONE', #2751, 23.85284712729792389, 0.9599310885968833640 ) ;
#15004=CARTESIAN_POINT ( 'NONE',  ( 0.000000000000000000, 23.00000000000000000, 0.000000000000000000 ) ) ;
#15006=CARTESIAN_POINT ( 'NONE',  ( 0.000000000000000000, 36.00000000000000000, 0.000000000000000000 ) ) ;
#15035=CARTESIAN_POINT ( 'NONE',  ( -13.14518615778179900, 38.12265625108393152, -5.444914386472297529 ) ) ;
#15041=EDGE_LOOP ( 'NONE', ( #4862, #9091, #8003, #19956 ) ) ;
#15064=CARTESIAN_POINT ( 'NONE',  ( 2.493653234604083739E-15, 32.56640625216787299, 13.57481594606304576 ) ) ;
#15065=CARTESIAN_POINT ( 'NONE',  ( -13.57481594606304753, 37.77539062499999289, -5.622872871577873077 ) ) ;
#15066=CARTESIAN_POINT ( 'NONE',  ( 9.295050272127047819, 38.66835937608393436, 9.295050272127046043 ) ) ;
#15084=EDGE_LOOP ( 'NONE', ( #27858, #14261, #27557, #6225 ) ) ;
#15089=CARTESIAN_POINT ( 'NONE',  ( -9.295050272127044266, 34.50117187608393721, 9.295050272127047819 ) ) ;
#15090=CARTESIAN_POINT ( 'NONE',  ( -5.444914386472297529, 40.60312500108393863, -13.14518615778179900 ) ) ;
#15107=CARTESIAN_POINT ( 'NONE',  ( -9.295050272127044266, 33.50898437608393010, 9.295050272127047819 ) ) ;
#15115=FACE_OUTER_BOUND ( 'NONE', #11223, .T. ) ;
#15117=ORIENTED_EDGE ( 'NONE', *, *, #984, .T. ) ;
#15118=DIRECTION ( 'NONE',  ( 0.000000000000000000, 0.000000000000000000, -1.000000000000000000 ) ) ;
#15123=CARTESIAN_POINT ( 'NONE',  ( -5.444914386472299306, 38.32109375108394289, 13.14518615778179722 ) ) ;
#15127=CARTESIAN_POINT ( 'NONE',  ( 0.000000000000000000, 1.500000000000001332, 0.000000000000000000 ) ) ;
#15131=VERTEX_POINT ( 'NONE', #365 ) ;
#15134=ORIENTED_EDGE ( 'NONE', *, *, #10867, .T. ) ;
#15143=CYLINDRICAL_SURFACE ( 'NONE', #3668, 23.00000000000001421 ) ;
#15159=CARTESIAN_POINT ( 'NONE',  ( 9.295050272127047819, 32.31835937608393294, 9.295050272127046043 ) ) ;
#15173=CARTESIAN_POINT ( 'NONE',  ( 13.14518615778179900, 38.61875000108393152, -5.444914386472297529 ) ) ;
#15203=CARTESIAN_POINT ( 'NONE',  ( 5.622872871577871301, 38.37070312499999147, -13.57481594606304753 ) ) ;
#15205=CARTESIAN_POINT ( 'NONE',  ( -8.049105076161786076E-16, 38.17226562608394147, -13.14518615778179544 ) ) ;
#15228=ORIENTED_EDGE ( 'NONE', *, *, #3794, .T. ) ;
#15233=CARTESIAN_POINT ( 'NONE',  ( 9.295050272127046043, 38.86679687608393863, -9.295050272127046043 ) ) ;
#15267=CARTESIAN_POINT ( 'NONE',  ( -13.14518615778179900, 39.71015625108393010, -5.444914386472297529 ) ) ;
#15283=CIRCLE ( 'NONE', #18944, 1.000000000000000888 ) ;
#15319=CARTESIAN_POINT ( 'NONE',  ( 13.14518615778179900, 40.10703125108393152, 5.444914386472293977 ) ) ;
#15345=ORIENTED_EDGE ( 'NONE', *, *, #1518, .T. ) ;
#15348=CARTESIAN_POINT ( 'NONE',  ( 13.57481594606304753, 37.47773437500001137, -5.622872871577873077 ) ) ;
#15349=CARTESIAN_POINT ( 'NONE',  ( 2.007297010069739596, 35.99999999999998579, -13.40042260803723373 ) ) ;
#15350=CARTESIAN_POINT ( 'NONE',  ( -13.14518615778179544, 38.37070312608393152, 0.000000000000000000 ) ) ;
#15360=CARTESIAN_POINT ( 'NONE',  ( 3.061616997868384226E-15, 23.00000000000000000, 25.00000000000001066 ) ) ;
#15377=CARTESIAN_POINT ( 'NONE',  ( 13.14518615778179722, 32.46718750108393436, -5.444914386472297529 ) ) ;
#15378=CARTESIAN_POINT ( 'NONE',  ( -5.444914386472297529, 39.01562500108394005, -13.14518615778179900 ) ) ;
#15381=CARTESIAN_POINT ( 'NONE',  ( -13.57481594606304398, 32.31835937499999289, 5.622872871577880183 ) ) ;
#15410=VERTEX_POINT ( 'NONE', #6872 ) ;
#15412=CARTESIAN_POINT ( 'NONE',  ( -8.049105076161786076E-16, 38.76757812608393294, -13.14518615778179544 ) ) ;
#15433=LINE ( 'NONE', #17729, #19845 ) ;
#15450=DIRECTION ( 'NONE',  ( 0.000000000000000000, 1.000000000000000000, 0.000000000000000000 ) ) ;
#15462=CARTESIAN_POINT ( 'NONE',  ( -5.444914386472297529, 38.81718750108393579, -13.14518615778179900 ) ) ;
#15479=CIRCLE ( 'NONE', #3195, 1.000000000000000888 ) ;
#15481=CARTESIAN_POINT ( 'NONE',  ( 13.01985494039077729, 35.99999999999995026, 3.369129453355339976 ) ) ;
#15492=CARTESIAN_POINT ( 'NONE',  ( 6.944426393311537993, 31.75150625057403175, -11.16113171639042356 ) ) ;
#15495=CARTESIAN_POINT ( 'NONE',  ( -13.57481594606304576, 37.03124999999999289, 0.000000000000000000 ) ) ;
#15497=CARTESIAN_POINT ( 'NONE',  ( 5.444914386472302859, 37.82500000108392868, 13.14518615778179189 ) ) ;
#15524=CARTESIAN_POINT ( 'NONE',  ( -13.14518615778179189, 32.86406250108393579, 5.444914386472304635 ) ) ;
#15525=CARTESIAN_POINT ( 'NONE',  ( -13.14518615778179189, 40.00781250108393294, 5.444914386472304635 ) ) ;
#15556=CARTESIAN_POINT ( 'NONE',  ( -5.444914386472299306, 39.90859375108393436, 13.14518615778179722 ) ) ;
#15603=ORIENTED_EDGE ( 'NONE', *, *, #26376, .T. ) ;
#15609=CARTESIAN_POINT ( 'NONE',  ( 13.14518615778179900, 36.93203125108394147, 5.444914386472293977 ) ) ;
#15636=CARTESIAN_POINT ( 'NONE',  ( 9.598844408820459861, 39.80937500216786873, 9.598844408820456309 ) ) ;
#15644=CARTESIAN_POINT ( 'NONE',  ( -9.598844408820454532, 38.71796874999999716, 9.598844408820459861 ) ) ;
#15646=CARTESIAN_POINT ( 'NONE',  ( -8.049105076161786076E-16, 34.20351562608394147, -13.14518615778179544 ) ) ;
#15660=CARTESIAN_POINT ( 'NONE',  ( 5.622872871577878406, 34.89804687499999147, 13.57481594606304398 ) ) ;
#15670=ORIENTED_EDGE ( 'NONE', *, *, #3745, .T. ) ;
#15672=CARTESIAN_POINT ( 'NONE',  ( -9.295050272127046043, 37.47773437608393010, -9.295050272127046043 ) ) ;
#15699=ADVANCED_FACE ( 'NONE', ( #9508 ), #18769, .T. ) ;
#15702=VECTOR ( 'NONE', #21375, 1000.000000000000000 ) ;
#15703=CARTESIAN_POINT ( 'NONE',  ( -13.14518615778179900, 38.12265625108393152, -5.444914386472297529 ) ) ;
#15725=VERTEX_POINT ( 'NONE', #15908 ) ;
#15751=CARTESIAN_POINT ( 'NONE',  ( 9.295050272127046043, 35.49335937608393010, -9.295050272127046043 ) ) ;
#15771=AXIS2_PLACEMENT_3D ( 'NONE', #908, #15450, #9862 ) ;
#15774=CARTESIAN_POINT ( 'NONE',  ( 13.57481594606304931, 39.85898437716787157, 5.622872871577869525 ) ) ;
#15780=DIRECTION ( 'NONE',  ( -0.000000000000000000, -1.000000000000000000, -0.000000000000000000 ) ) ;
#15783=CARTESIAN_POINT ( 'NONE',  ( -5.622872871577873077, 35.29492187500000000, -13.57481594606304753 ) ) ;
#15787=CARTESIAN_POINT ( 'NONE',  ( 5.444914386472297529, 35.74140625108393721, -13.14518615778179900 ) ) ;
#15789=CARTESIAN_POINT ( 'NONE',  ( -9.295050272127046043, 35.69179687608393436, -9.295050272127046043 ) ) ;
#15790=CARTESIAN_POINT ( 'NONE',  ( -13.57481594606304576, 36.38632812716788578, 5.622872871577880183 ) ) ;
#15799=ORIENTED_EDGE ( 'NONE', *, *, #19418, .T. ) ;
#15812=VERTEX_POINT ( 'NONE', #5576 ) ;
#15813=CARTESIAN_POINT ( 'NONE',  ( -13.14518615778179900, 37.52734375108393294, -5.444914386472297529 ) ) ;
#15828=CARTESIAN_POINT ( 'NONE',  ( 0.000000000000000000, 36.00000000000000000, 0.000000000000000000 ) ) ;
#15841=CARTESIAN_POINT ( 'NONE',  ( 5.444914386472302859, 35.24531250108393010, 13.14518615778179189 ) ) ;
#15854=VERTEX_POINT ( 'NONE', #12091 ) ;
#15862=CARTESIAN_POINT ( 'NONE',  ( -8.312177448680279460E-16, 34.45156249999999432, -13.57481594606304576 ) ) ;
#15881=( GEOMETRIC_REPRESENTATION_CONTEXT ( 3 ) GLOBAL_UNCERTAINTY_ASSIGNED_CONTEXT ( ( #2155 ) ) GLOBAL_UNIT_ASSIGNED_CONTEXT ( ( #19187, #16901, #27888 ) ) REPRESENTATION_CONTEXT ( 'NONE', 'WORKASPACE' ) );
#15888=CARTESIAN_POINT ( 'NONE',  ( -9.295050272127044266, 36.68398437608392726, 9.295050272127047819 ) ) ;
#15907=CARTESIAN_POINT ( 'NONE',  ( -13.57481594606304576, 40.30546875216787583, 0.000000000000000000 ) ) ;
#15908=CARTESIAN_POINT ( 'NONE',  ( -2.655063156357168549E-15, 10.00000000000000000, -19.22649730810373470 ) ) ;
#15918=CARTESIAN_POINT ( 'NONE',  ( 2.493653234604083739E-15, 33.26093749999999716, 13.57481594606304576 ) ) ;
#15920=CARTESIAN_POINT ( 'NONE',  ( -13.14518615778179189, 35.24531250108393721, 5.444914386472304635 ) ) ;
#15923=CARTESIAN_POINT ( 'NONE',  ( -9.598844408820458085, 35.44375000216787441, -9.598844408820458085 ) ) ;
#15949=CARTESIAN_POINT ( 'NONE',  ( -13.14518615778179544, 35.19570312608393436, 0.000000000000000000 ) ) ;
#15981=CARTESIAN_POINT ( 'NONE',  ( 9.295050272127046043, 36.28710937608393294, -9.295050272127046043 ) ) ;
#16008=ORIENTED_EDGE ( 'NONE', *, *, #88, .T. ) ;
#16020=CARTESIAN_POINT ( 'NONE',  ( -13.57481594606304398, 34.00507812716787726, 5.622872871577880183 ) ) ;
#16027=DIRECTION ( 'NONE',  ( 0.000000000000000000, 0.000000000000000000, -1.000000000000000000 ) ) ;
#16028=CARTESIAN_POINT ( 'NONE',  ( 13.14518615778179900, 37.03125000108393294, -5.444914386472297529 ) ) ;
#16029=CYLINDRICAL_SURFACE ( 'NONE', #13314, 25.00000000000001066 ) ;
#16047=PRODUCT ( 'Suction Cups Set (x4)', 'Suction Cups Set (x4)', '', ( #21235 ) ) ;
#16051=CARTESIAN_POINT ( 'NONE',  ( -9.295050272127046043, 32.71523437608393436, -9.295050272127046043 ) ) ;
#16055=CARTESIAN_POINT ( 'NONE',  ( 13.57481594606304931, 39.06523437716786873, 5.622872871577869525 ) ) ;
#16058=CARTESIAN_POINT ( 'NONE',  ( -13.57481594606304753, 33.11210937716787583, -5.622872871577872189 ) ) ;
#16064=CARTESIAN_POINT ( 'NONE',  ( -13.57481594606304753, 35.39414062499999147, -5.622872871577873077 ) ) ;
#16066=CARTESIAN_POINT ( 'NONE',  ( -5.444914386472297529, 35.04687500108393294, -13.14518615778179900 ) ) ;
#16069=CARTESIAN_POINT ( 'NONE',  ( 9.598844408820456309, 37.62656250216787157, -9.598844408820458085 ) ) ;
#16080=LINE ( 'NONE', #16232, #21689 ) ;
#16092=ORIENTED_EDGE ( 'NONE', *, *, #27642, .T. ) ;
#16093=CARTESIAN_POINT ( 'NONE',  ( 9.295050272127046043, 34.89804687608393863, -9.295050272127046043 ) ) ;
#16095=EDGE_CURVE ( 'NONE', #25525, #15131, #794, .T. ) ;
#16118=CARTESIAN_POINT ( 'NONE',  ( 0.000000000000000000, 23.00000000000000000, 0.000000000000000000 ) ) ;
#16127=CARTESIAN_POINT ( 'NONE',  ( -9.295050272127044266, 35.89023437608393152, 9.295050272127047819 ) ) ;
#16133=CIRCLE ( 'NONE', #23866, 13.57481594606304576 ) ;
#16140=LINE ( 'NONE', #18433, #7573 ) ;
#16177=DIRECTION ( 'NONE',  ( 0.000000000000000000, 0.000000000000000000, -1.000000000000000000 ) ) ;
#16182=MECHANICAL_DESIGN_GEOMETRIC_PRESENTATION_REPRESENTATION('',(#7058),#2989);
#16198=CARTESIAN_POINT ( 'NONE',  ( 2.414731522848535132E-15, 33.80664062608393294, 13.14518615778179544 ) ) ;
#16201=CARTESIAN_POINT ( 'NONE',  ( -13.57481594606304753, 39.46210937716787726, -5.622872871577873077 ) ) ;
#16205=CARTESIAN_POINT ( 'NONE',  ( -5.622872871577873966, 33.01289062716787726, -13.57481594606304753 ) ) ;
#16211=CARTESIAN_POINT ( 'NONE',  ( 5.622872871577871301, 34.40195312499999858, -13.57481594606304753 ) ) ;
#16214=CARTESIAN_POINT ( 'NONE',  ( -13.14518615778179189, 34.45156250108394147, 5.444914386472304635 ) ) ;
#16217=CARTESIAN_POINT ( 'NONE',  ( -13.57481594606304576, 36.33671875216787583, 0.000000000000000000 ) ) ;
#16222=CARTESIAN_POINT ( 'NONE',  ( 5.622872871578015186, 34.99726562716787015, 13.57481594606290543 ) ) ;
#16232=CARTESIAN_POINT ( 'NONE',  ( 7.171391131791534868, 31.93754143773660203, -11.52591762960188149 ) ) ;
#16244=CARTESIAN_POINT ( 'NONE',  ( -13.14518615778179189, 36.03906250108394005, 5.444914386472304635 ) ) ;
#16262=CARTESIAN_POINT ( 'NONE',  ( 0.000000000000000000, 0.000000000000000000, 0.000000000000000000 ) ) ;
#16274=CARTESIAN_POINT ( 'NONE',  ( -5.444914386472297529, 36.43593750108392726, -13.14518615778179900 ) ) ;
#16277=ADVANCED_FACE ( 'NONE', ( #26635 ), #19623, .T. ) ;
#16297=CARTESIAN_POINT ( 'NONE',  ( 9.598844408820456309, 32.07031250216787299, -9.598844408820458085 ) ) ;
#16322=DIRECTION ( 'NONE',  ( -0.000000000000000000, -1.000000000000000000, -0.000000000000000000 ) ) ;
#16328=CARTESIAN_POINT ( 'NONE',  ( 9.295050272127047819, 39.46210937608393721, 9.295050272127046043 ) ) ;
#16347=( NAMED_UNIT ( * ) PLANE_ANGLE_UNIT ( ) SI_UNIT ( $, .RADIAN. ) );
#16356=CARTESIAN_POINT ( 'NONE',  ( -13.57481594606304753, 34.60039062499999574, -5.622872871577873077 ) ) ;
#16358=CARTESIAN_POINT ( 'NONE',  ( 9.598844408820459861, 39.71015624999999716, 9.598844408820456309 ) ) ;
#16360=CARTESIAN_POINT ( 'NONE',  ( -5.444914386472299306, 34.35234375108392868, 13.14518615778179722 ) ) ;
#16361=CARTESIAN_POINT ( 'NONE',  ( 9.598844408820456309, 36.03906250216787299, -9.598844408820458085 ) ) ;
#16372=DIRECTION ( 'NONE',  ( 0.000000000000000000, 1.000000000000000000, 0.000000000000000000 ) ) ;
#16384=CARTESIAN_POINT ( 'NONE',  ( 9.295050272127047819, 33.90585937608393863, 9.295050272127046043 ) ) ;
#16397=CARTESIAN_POINT ( 'NONE',  ( -13.57481594606304753, 33.01289062499999716, -5.622872871577872189 ) ) ;
#16416=CARTESIAN_POINT ( 'NONE',  ( 9.295050272127047819, 33.70742187608393436, 9.295050272127046043 ) ) ;
#16463=CARTESIAN_POINT ( 'NONE',  ( -9.295050272127044266, 40.05742187608393579, 9.295050272127047819 ) ) ;
#16470=ORIENTED_EDGE ( 'NONE', *, *, #27168, .F. ) ;
#16485=SURFACE_STYLE_USAGE ( .BOTH. , #5532 ) ;
#16486=DIRECTION ( 'NONE',  ( 0.000000000000000000, 0.000000000000000000, -1.000000000000000000 ) ) ;
#16497=CARTESIAN_POINT ( 'NONE',  ( -10.54595693695916125, 36.00000000000001421, -8.172591659953413412 ) ) ;
#16498=CARTESIAN_POINT ( 'NONE',  ( 5.622872871577878406, 39.66054687500000142, 13.57481594606304576 ) ) ;
#16500=CARTESIAN_POINT ( 'NONE',  ( -9.295050272127046043, 33.31054687608393294, -9.295050272127046043 ) ) ;
#16501=EDGE_CURVE ( 'NONE', #19839, #26327, #3765, .T. ) ;
#16503=CARTESIAN_POINT ( 'NONE',  ( -9.598844408820454532, 33.26093750216787726, 9.598844408820459861 ) ) ;
#16523=VECTOR ( 'NONE', #24456, 1000.000000000000000 ) ;
#16526=CARTESIAN_POINT ( 'NONE',  ( -5.444914386472299306, 34.55078125108393294, 13.14518615778179722 ) ) ;
#16556=ORIENTED_EDGE ( 'NONE', *, *, #7420, .T. ) ;
#16558=CARTESIAN_POINT ( 'NONE',  ( -13.14518615778179544, 33.40976562608393863, 0.000000000000000000 ) ) ;
#16570=CARTESIAN_POINT ( 'NONE',  ( -13.14518615778179544, 37.37851562608393863, 0.000000000000000000 ) ) ;
#16601=CARTESIAN_POINT ( 'NONE',  ( 2.493653234604083739E-15, 33.36015625216786873, 13.57481594606304576 ) ) ;
#16605=CARTESIAN_POINT ( 'NONE',  ( 2.414731522848535132E-15, 40.15664062608393436, 13.14518615778179544 ) ) ;
#16607=VECTOR ( 'NONE', #27776, 1000.000000000000114 ) ;
#16628=DIRECTION ( 'NONE',  ( 0.000000000000000000, -0.000000000000000000, 1.000000000000000000 ) ) ;
#16635=CARTESIAN_POINT ( 'NONE',  ( -5.622872871577873077, 32.11992187499999574, -13.57481594606304753 ) ) ;
#16638=EDGE_LOOP ( 'NONE', ( #5929, #14575, #4574, #13968 ) ) ;
#16639=CARTESIAN_POINT ( 'NONE',  ( -8.049105076161786076E-16, 32.61601562608393579, -13.14518615778179544 ) ) ;
#16640=CARTESIAN_POINT ( 'NONE',  ( 9.295050272127046043, 32.31835937608393294, -9.295050272127046043 ) ) ;
#16641=CARTESIAN_POINT ( 'NONE',  ( -5.622872871577873077, 31.72304687716787441, 13.57481594606304753 ) ) ;
#16657=ADVANCED_FACE ( 'NONE', ( #16861 ), #13692, .T. ) ;
#16666=CARTESIAN_POINT ( 'NONE',  ( -9.295050272127046043, 32.71523437608393436, -9.295050272127046043 ) ) ;
#16668=CARTESIAN_POINT ( 'NONE',  ( 0.000000000000000000, 20.00000000000000000, 0.000000000000000000 ) ) ;
#16672=CYLINDRICAL_SURFACE ( 'NONE', #8758, 13.57481594606304576 ) ;
#16685=ORIENTED_EDGE ( 'NONE', *, *, #22385, .T. ) ;
#16696=CARTESIAN_POINT ( 'NONE',  ( -8.049105076161786076E-16, 32.41757812608393863, -13.14518615778179544 ) ) ;
#16701=AXIS2_PLACEMENT_3D ( 'NONE', #27970, #25678, #8428 ) ;
#16713=CARTESIAN_POINT ( 'NONE',  ( 2.414731522848535132E-15, 32.81445312608393294, 13.14518615778179544 ) ) ;
#16717=LINE ( 'NONE', #19133, #23637 ) ;
#16721=CARTESIAN_POINT ( 'NONE',  ( 9.598844408820459861, 31.87187500216787228, 9.598844408820456309 ) ) ;
#16755=CARTESIAN_POINT ( 'NONE',  ( -2.955559473995892819E-15, 1.500000000000001332, -24.13397459621556607 ) ) ;
#16774=CARTESIAN_POINT ( 'NONE',  ( 13.57481594606304931, 38.96601562499999005, 5.622872871577869525 ) ) ;
#16776=CARTESIAN_POINT ( 'NONE',  ( 2.493653234604083739E-15, 33.36015625216786873, 13.57481594606304576 ) ) ;
#16796=ORIENTED_EDGE ( 'NONE', *, *, #11414, .T. ) ;
#16800=CARTESIAN_POINT ( 'NONE',  ( -8.049105076161786076E-16, 34.20351562608394147, -13.14518615778179544 ) ) ;
#16815=EDGE_CURVE ( 'NONE', #19989, #18417, #2783, .T. ) ;
#16820=CARTESIAN_POINT ( 'NONE',  ( 0.7050241099688876467, 36.00000000000002842, 13.13343125082108820 ) ) ;
#16826=CARTESIAN_POINT ( 'NONE',  ( -5.622872871577873966, 31.42539062716787157, -13.57481594606304753 ) ) ;
#16828=EDGE_CURVE ( 'NONE', #18529, #4666, #17066, .T. ) ;
#16834=CARTESIAN_POINT ( 'NONE',  ( -9.295050272127044266, 33.50898437608393010, 9.295050272127047819 ) ) ;
#16841=ORIENTED_EDGE ( 'NONE', *, *, #571, .F. ) ;
#16848=CARTESIAN_POINT ( 'NONE',  ( -9.295050272127044266, 31.92148437608393508, 9.295050272127047819 ) ) ;
#16861=FACE_OUTER_BOUND ( 'NONE', #13404, .T. ) ;
#16863=ORIENTED_EDGE ( 'NONE', *, *, #11904, .F. ) ;
#16871=MANIFOLD_SOLID_BREP ( 'Cavity1', #26271 ) ;
#16890=ORIENTED_EDGE ( 'NONE', *, *, #23765, .T. ) ;
#16901=( NAMED_UNIT ( * ) PLANE_ANGLE_UNIT ( ) SI_UNIT ( $, .RADIAN. ) );
#16906=CARTESIAN_POINT ( 'NONE',  ( -9.295050272127046043, 31.92148437608393508, -9.295050272127046043 ) ) ;
#16907=CARTESIAN_POINT ( 'NONE',  ( 13.14518615778179544, 33.01289062608393010, -1.609821015232357215E-15 ) ) ;
#16908=CARTESIAN_POINT ( 'NONE',  ( -5.622872871577873077, 34.10429687716786873, 13.57481594606304753 ) ) ;
#16928=ORIENTED_EDGE ( 'NONE', *, *, #6682, .T. ) ;
#16945=CARTESIAN_POINT ( 'NONE',  ( -12.83975123685816833, 36.00000000000000000, 2.850296047819892209 ) ) ;
#16952=ORIENTED_EDGE ( 'NONE', *, *, #14397, .T. ) ;
#16961=ORIENTED_EDGE ( 'NONE', *, *, #22061, .F. ) ;
#16962=CARTESIAN_POINT ( 'NONE',  ( 5.444914386472302859, 35.44375000108393436, 13.14518615778179189 ) ) ;
#16963=CARTESIAN_POINT ( 'NONE',  ( -5.444914386472297529, 32.46718750108393436, -13.14518615778179900 ) ) ;
#16981=CARTESIAN_POINT ( 'NONE',  ( -9.295050272127046043, 31.72304687608393081, -9.295050272127046043 ) ) ;
#17007=CARTESIAN_POINT ( 'NONE',  ( 9.598844408820459861, 33.45937500216787441, 9.598844408820456309 ) ) ;
#17016=AXIS2_PLACEMENT_3D ( 'NONE', #2039, #9009, #11122 ) ;
#17035=CIRCLE ( 'NONE', #8400, 19.22649730810373470 ) ;
#17036=( NAMED_UNIT ( * ) PLANE_ANGLE_UNIT ( ) SI_UNIT ( $, .RADIAN. ) );
#17042=CARTESIAN_POINT ( 'NONE',  ( 2.414731522848535132E-15, 32.02070312608393010, 13.14518615778179544 ) ) ;
#17043=CARTESIAN_POINT ( 'NONE',  ( 5.444914386472297529, 39.51171875108392584, -13.14518615778179900 ) ) ;
#17059=AXIS2_PLACEMENT_3D ( 'NONE', #4173, #6033, #17125 ) ;
#17066=CIRCLE ( 'NONE', #1183, 24.13397459621556962 ) ;
#17071=FACE_OUTER_BOUND ( 'NONE', #7492, .T. ) ;
#17078=EDGE_CURVE ( 'NONE', #8637, #17432, #22282, .T. ) ;
#17090=LINE ( 'NONE', #12388, #12015 ) ;
#17092=CARTESIAN_POINT ( 'NONE',  ( 0.000000000000000000, 23.00000000000000000, -25.00000000000001066 ) ) ;
#17094=ORIENTED_EDGE ( 'NONE', *, *, #17152, .T. ) ;
#17098=CARTESIAN_POINT ( 'NONE',  ( 13.14518615778179544, 35.59257812608393579, -1.609821015232357215E-15 ) ) ;
#17099=CARTESIAN_POINT ( 'NONE',  ( -9.295050272127046043, 38.27148437608393294, -9.295050272127046043 ) ) ;
#17125=DIRECTION ( 'NONE',  ( 0.000000000000000000, 0.000000000000000000, -1.000000000000000000 ) ) ;
#17128=CARTESIAN_POINT ( 'NONE',  ( 3.878385297391210518, 32.03609435653363136, -13.57481594606304576 ) ) ;
#17130=CIRCLE ( 'NONE', #28075, 13.57481594606304576 ) ;
#17152=EDGE_CURVE ( 'NONE', #22143, #26327, #11420, .T. ) ;
#17186=CARTESIAN_POINT ( 'NONE',  ( 13.14518615778179544, 37.77539062608393294, -1.609821015232357215E-15 ) ) ;
#17204=CARTESIAN_POINT ( 'NONE',  ( 10.56308295036056677, 36.00000000000000711, 8.196709705856857653 ) ) ;
#17214=CARTESIAN_POINT ( 'NONE',  ( 5.622872871577694553, 35.69179687499999432, 13.57481594606322695 ) ) ;
#17217=CARTESIAN_POINT ( 'NONE',  ( -9.295050272127046043, 36.68398437608393436, -9.295050272127046043 ) ) ;
#17226=CARTESIAN_POINT ( 'NONE',  ( -3.136173621347420060, 36.00000000000000711, 12.79489613812762450 ) ) ;
#17243=CARTESIAN_POINT ( 'NONE',  ( -13.14518615778179722, 35.93984375108393436, -5.444914386472297529 ) ) ;
#17244=CARTESIAN_POINT ( 'NONE',  ( 9.295050272127047819, 39.46210937608393721, 9.295050272127046043 ) ) ;
#17253=( GEOMETRIC_REPRESENTATION_CONTEXT ( 3 ) GLOBAL_UNCERTAINTY_ASSIGNED_CONTEXT ( ( #19814 ) ) GLOBAL_UNIT_ASSIGNED_CONTEXT ( ( #13163, #17036, #10478 ) ) REPRESENTATION_CONTEXT ( 'NONE', 'WORKASPACE' ) );
#17264=CARTESIAN_POINT ( 'NONE',  ( -13.14518615778179544, 32.61601562608393579, 0.000000000000000000 ) ) ;
#17279=CARTESIAN_POINT ( 'NONE',  ( 5.444914386472302859, 38.42031250108393436, 13.14518615778179189 ) ) ;
#17283=DIRECTION ( 'NONE',  ( 0.000000000000000000, 1.000000000000000000, 0.000000000000000000 ) ) ;
#17315=CARTESIAN_POINT ( 'NONE',  ( 13.14518615778179900, 33.26093750108393721, -5.444914386472297529 ) ) ;
#17324=CIRCLE ( 'NONE', #47, 23.26794919243112858 ) ;
#17325=CARTESIAN_POINT ( 'NONE',  ( 0.000000000000000000, 36.00000000000000000, -13.57481594606304576 ) ) ;
#17332=CARTESIAN_POINT ( 'NONE',  ( 13.14518615778179900, 40.20625000108393010, -5.444914386472297529 ) ) ;
#17349=CARTESIAN_POINT ( 'NONE',  ( 13.24545034676895305, 36.00000000000001421, 2.307131236159923215 ) ) ;
#17361=CARTESIAN_POINT ( 'NONE',  ( 9.598844408820459861, 35.74140624999999716, 9.598844408820456309 ) ) ;
#17363=CARTESIAN_POINT ( 'NONE',  ( -13.14518615778179900, 35.93984375108393436, -5.444914386472297529 ) ) ;
#17386=ORIENTED_EDGE ( 'NONE', *, *, #6000, .F. ) ;
#17388=CARTESIAN_POINT ( 'NONE',  ( -13.14518615778179900, 39.90859375108394147, -5.444914386472297529 ) ) ;
#17421=CARTESIAN_POINT ( 'NONE',  ( -5.444914386472297529, 39.61093750108393152, -13.14518615778179900 ) ) ;
#17432=VERTEX_POINT ( 'NONE', #11528 ) ;
#17455=DIRECTION ( 'NONE',  ( 0.000000000000000000, 1.000000000000000000, 0.000000000000000000 ) ) ;
#17466=CARTESIAN_POINT ( 'NONE',  ( -8.049105076161786076E-16, 39.56132812608393579, -13.14518615778179544 ) ) ;
#17491=CONICAL_SURFACE ( 'NONE', #8851, 25.00000000000001066, 0.9599310885968833640 ) ;
#17499=CARTESIAN_POINT ( 'NONE',  ( -8.312177448680279460E-16, 37.62656249999999858, -13.57481594606304576 ) ) ;
#17501=CARTESIAN_POINT ( 'NONE',  ( -5.444914386472297529, 38.22187500108393010, -13.14518615778179900 ) ) ;
#17525=CARTESIAN_POINT ( 'NONE',  ( 5.622872871577870413, 32.91367187716787157, -13.57481594606304753 ) ) ;
#17528=CARTESIAN_POINT ( 'NONE',  ( -13.14518615778179544, 35.19570312608393436, 0.000000000000000000 ) ) ;
#17529=CARTESIAN_POINT ( 'NONE',  ( -9.295050272127044266, 38.46992187608393721, 9.295050272127047819 ) ) ;
#17562=CARTESIAN_POINT ( 'NONE',  ( 13.14518615778179900, 40.20625000108393010, -5.444914386472297529 ) ) ;
#17599=ADVANCED_FACE ( 'NONE', ( #14201 ), #7223, .F. ) ;
#17608=CARTESIAN_POINT ( 'NONE',  ( 9.295050272127047819, 40.05742187608392868, 9.295050272127046043 ) ) ;
#17615=DIRECTION ( 'NONE',  ( -0.000000000000000000, -1.000000000000000000, -0.000000000000000000 ) ) ;
#17627=CARTESIAN_POINT ( 'NONE',  ( 9.031440422455050410, 35.99999999999997868, 9.765766397118351705 ) ) ;
#17633=VECTOR ( 'NONE', #11981, 1000.000000000000000 ) ;
#17641=CARTESIAN_POINT ( 'NONE',  ( -13.57481594606304753, 36.18789062499999432, -5.622872871577873077 ) ) ;
#17642=CARTESIAN_POINT ( 'NONE',  ( -0.9955612250524552564, 35.99999999999999289, -13.45766439703027118 ) ) ;
#17643=CARTESIAN_POINT ( 'NONE',  ( 5.444914386472297529, 37.32890625108393579, -13.14518615778179900 ) ) ;
#17669=CARTESIAN_POINT ( 'NONE',  ( 13.14518615778179544, 32.41757812608393863, -1.609821015232357215E-15 ) ) ;
#17671=CARTESIAN_POINT ( 'NONE',  ( 9.295050272127046043, 40.45429687608393721, -9.295050272127046043 ) ) ;
#17683=CARTESIAN_POINT ( 'NONE',  ( -5.622872871577873966, 34.79882812499999289, 13.57481594606304753 ) ) ;
#17684=EDGE_CURVE ( 'NONE', #25472, #25494, #4221, .T. ) ;
#17709=CARTESIAN_POINT ( 'NONE',  ( 13.14518615778179544, 40.15664062608393436, -1.609821015232357215E-15 ) ) ;
#17710=COLOUR_RGB ( '', 0.40784314, 0.44705882, 0.49803922) ;
#17729=CARTESIAN_POINT ( 'NONE',  ( 0.000000000000000000, 36.00000000000000000, -13.57481594606304576 ) ) ;
#17736=ORIENTED_EDGE ( 'NONE', *, *, #3875, .F. ) ;
#17759=CARTESIAN_POINT ( 'NONE',  ( 13.14518615778179900, 36.13828125108393863, 5.444914386472293977 ) ) ;
#17770=CARTESIAN_POINT ( 'NONE',  ( 9.598844408820459861, 33.36015624999999574, 9.598844408820456309 ) ) ;
#17782=CARTESIAN_POINT ( 'NONE',  ( 13.57481594606304753, 38.37070312716786447, -5.622872871577873077 ) ) ;
#17789=CARTESIAN_POINT ( 'NONE',  ( 13.57481594606304576, 35.84062499999999574, -1.662435489736055892E-15 ) ) ;
#17792=CARTESIAN_POINT ( 'NONE',  ( 13.14518615778179900, 37.92421875108392726, 5.444914386472293977 ) ) ;
#17812=EDGE_LOOP ( 'NONE', ( #12485, #16092, #12936, #18654, #5531, #20027, #27363, #24548, #11760, #15117, #9824, #5865, #14953, #1620 ) ) ;
#17816=CARTESIAN_POINT ( 'NONE',  ( -8.049105076161786076E-16, 35.79101562608394005, -13.14518615778179544 ) ) ;
#17821=ORIENTED_EDGE ( 'NONE', *, *, #23765, .F. ) ;
#17836=ORIENTED_EDGE ( 'NONE', *, *, #14737, .F. ) ;
#17851=EDGE_CURVE ( 'NONE', #3596, #9781, #11325, .T. ) ;
#17860=DIRECTION ( 'NONE',  ( 0.000000000000000000, 0.000000000000000000, 1.000000000000000000 ) ) ;
#17891=ORIENTED_EDGE ( 'NONE', *, *, #19264, .F. ) ;
#17897=CARTESIAN_POINT ( 'NONE',  ( -13.14518615778179900, 37.32890625108393579, -5.444914386472297529 ) ) ;
#17920=CARTESIAN_POINT ( 'NONE',  ( 9.598844408820456309, 39.21406250216787015, -9.598844408820458085 ) ) ;
#17926=CARTESIAN_POINT ( 'NONE',  ( 2.493653234604083739E-15, 35.64218749999999147, 13.57481594606304576 ) ) ;
#17928=CARTESIAN_POINT ( 'NONE',  ( -5.622872871577873077, 36.88242187499999858, -13.57481594606304753 ) ) ;
#17930=CARTESIAN_POINT ( 'NONE',  ( -5.444914386472299306, 32.96328125108393436, 13.14518615778179722 ) ) ;
#17933=CARTESIAN_POINT ( 'NONE',  ( -9.598844408820454532, 37.22968750216787726, 9.598844408820459861 ) ) ;
#17956=CARTESIAN_POINT ( 'NONE',  ( -5.444914386472297529, 35.04687500108393294, -13.14518615778179900 ) ) ;
#17979=DIRECTION ( 'NONE',  ( -0.000000000000000000, -1.000000000000000000, -0.000000000000000000 ) ) ;
#17988=CARTESIAN_POINT ( 'NONE',  ( 9.295050272127046043, 37.08085937608393579, -9.295050272127046043 ) ) ;
#18025=CARTESIAN_POINT ( 'NONE',  ( -5.622872871577964560, 33.80664062716787299, -13.57481594606295339 ) ) ;
#18031=CARTESIAN_POINT ( 'NONE',  ( -8.312177448680279460E-16, 35.34453125216787583, -13.57481594606304576 ) ) ;
#18035=CARTESIAN_POINT ( 'NONE',  ( 13.14518615778179544, 34.60039062608392868, -1.609821015232357215E-15 ) ) ;
#18058=CARTESIAN_POINT ( 'NONE',  ( 5.622872871577871301, 39.26367187716787299, -13.57481594606304753 ) ) ;
#18066=CARTESIAN_POINT ( 'NONE',  ( 5.622872871577871301, 35.19570312499999432, -13.57481594606304753 ) ) ;
#18069=CARTESIAN_POINT ( 'NONE',  ( 5.444914386472302859, 35.44375000108393436, 13.14518615778179189 ) ) ;
#18071=CARTESIAN_POINT ( 'NONE',  ( -5.444914386472297529, 35.64218750108393152, -13.14518615778179722 ) ) ;
#18073=CARTESIAN_POINT ( 'NONE',  ( -5.622872871577873077, 36.98164062716787015, -13.57481594606304753 ) ) ;
#18098=CARTESIAN_POINT ( 'NONE',  ( 5.444914386472297529, 36.53515625108393294, -13.14518615778179900 ) ) ;
#18108=CARTESIAN_POINT ( 'NONE',  ( 0.000000000000000000, 36.00000000000000000, 0.000000000000000000 ) ) ;
#18121=CARTESIAN_POINT ( 'NONE',  ( 0.000000000000000000, 31.00000000000000000, 0.000000000000000000 ) ) ;
#18123=ADVANCED_FACE ( 'NONE', ( #7338 ), #2796, .T. ) ;
#18131=CARTESIAN_POINT ( 'NONE',  ( -13.14518615778179544, 38.17226562608393436, 0.000000000000000000 ) ) ;
#18166=VERTEX_POINT ( 'NONE', #3219 ) ;
#18172=DIRECTION ( 'NONE',  ( 6.123233995736778362E-17, 0.8660254037844380415, -0.5000000000000009992 ) ) ;
#18179=CARTESIAN_POINT ( 'NONE',  ( -9.598844408820454532, 35.64218750216787868, 9.598844408820459861 ) ) ;
#18182=CARTESIAN_POINT ( 'NONE',  ( -13.14518615778179900, 35.74140625108393721, -5.444914386472297529 ) ) ;
#18200=ADVANCED_FACE ( 'NONE', ( #20611 ), #3500, .F. ) ;
#18207=FACE_OUTER_BOUND ( 'NONE', #9187, .T. ) ;
#18211=EDGE_CURVE ( 'NONE', #1506, #8614, #4777, .T. ) ;
#18214=DIRECTION ( 'NONE',  ( 0.000000000000000000, 0.000000000000000000, -1.000000000000000000 ) ) ;
#18216=CARTESIAN_POINT ( 'NONE',  ( 13.57481594606304576, 34.25312499999999716, -1.662435489736055892E-15 ) ) ;
#18217=CARTESIAN_POINT ( 'NONE',  ( -13.14917398115171743, 36.00000000000000711, -1.058935892997135975 ) ) ;
#18219=CARTESIAN_POINT ( 'NONE',  ( -9.295050272127046043, 34.30273437608393294, -9.295050272127046043 ) ) ;
#18221=CARTESIAN_POINT ( 'NONE',  ( 9.295050272127046043, 34.69960937608393436, -9.295050272127046043 ) ) ;
#18222=EDGE_CURVE ( 'NONE', #27857, #27010, #23578, .T. ) ;
#18223=CARTESIAN_POINT ( 'NONE',  ( -8.312177448680279460E-16, 34.55078125216787299, -13.57481594606304576 ) ) ;
#18248=EDGE_LOOP ( 'NONE', ( #20605, #20448, #2237, #21985 ) ) ;
#18249=CARTESIAN_POINT ( 'NONE',  ( -8.049105076161786076E-16, 34.99726562608393721, -13.14518615778179544 ) ) ;
#18257=CARTESIAN_POINT ( 'NONE',  ( 2.493653234604083739E-15, 34.84843749999999574, 13.57481594606304576 ) ) ;
#18269=ORIENTED_EDGE ( 'NONE', *, *, #21043, .F. ) ;
#18270=( BOUNDED_CURVE ( )  B_SPLINE_CURVE ( 2, ( #149, #17525, #2851, #4564, #22099, #13225, #11520, #21957, #8977 ),
 .UNSPECIFIED., .F., .T. ) 
 B_SPLINE_CURVE_WITH_KNOTS ( ( 3, 2, 2, 2, 3 ),
 ( 0.7708333333333333703, 0.7812500000000000000, 0.7916666666666665186, 0.8020833333333332593, 0.8124999999999998890 ),
 .UNSPECIFIED. ) 
 CURVE ( )  GEOMETRIC_REPRESENTATION_ITEM ( )  RATIONAL_B_SPLINE_CURVE ( ( 1.000000000000000000, 0.9238795325112867385, 1.000000000000000000, 0.9238795325112867385, 1.000000000000000000, 0.9238795325112867385, 1.000000000000000000, 0.9238795325112875156, 0.9999999999999992228 ) ) 
 REPRESENTATION_ITEM ( '' )  );
#18271=DIRECTION ( 'NONE',  ( 0.000000000000000000, 0.000000000000000000, 1.000000000000000000 ) ) ;
#18281=CARTESIAN_POINT ( 'NONE',  ( 13.14518615778179900, 35.44375000108393436, -5.444914386472297529 ) ) ;
#18326=CARTESIAN_POINT ( 'NONE',  ( -13.57481594606304576, 35.54296875216788010, 0.000000000000000000 ) ) ;
#18331=DIRECTION ( 'NONE',  ( -6.123233995736778362E-17, -0.8660254037844380415, -0.5000000000000009992 ) ) ;
#18348=CARTESIAN_POINT ( 'NONE',  ( 3.755639919285892248, 31.78804746655075775, -13.14518615778179544 ) ) ;
#18350=CARTESIAN_POINT ( 'NONE',  ( 13.57481594606304576, 39.11484375216787157, -1.662435489736055892E-15 ) ) ;
#18358=CARTESIAN_POINT ( 'NONE',  ( -13.57481594606304576, 35.49335937499999005, 5.622872871577880183 ) ) ;
#18359=CARTESIAN_POINT ( 'NONE',  ( -12.56650672479864461, 36.00000000000000000, -4.295155080288879823 ) ) ;
#18360=CARTESIAN_POINT ( 'NONE',  ( 5.444914386472297529, 34.15390625108393863, -13.14518615778179900 ) ) ;
#18363=CARTESIAN_POINT ( 'NONE',  ( 9.295050272127047819, 34.50117187608393010, 9.295050272127046043 ) ) ;
#18364=CARTESIAN_POINT ( 'NONE',  ( -5.622872871577873077, 36.18789062716787441, -13.57481594606304753 ) ) ;
#18386=ORIENTED_EDGE ( 'NONE', *, *, #11414, .F. ) ;
#18389=CARTESIAN_POINT ( 'NONE',  ( -13.14518615778179189, 37.62656250108393863, 5.444914386472304635 ) ) ;
#18417=VERTEX_POINT ( 'NONE', #3325 ) ;
#18422=CARTESIAN_POINT ( 'NONE',  ( 9.295050272127047819, 36.08867187608392868, 9.295050272127046043 ) ) ;
#18433=CARTESIAN_POINT ( 'NONE',  ( 1.662435489736055892E-15, 36.00000000000000000, 13.57481594606304576 ) ) ;
#18468=VERTEX_POINT ( 'NONE', #12693 ) ;
#18490=EDGE_CURVE ( 'NONE', #15725, #5426, #5782, .T. ) ;
#18493=CARTESIAN_POINT ( 'NONE',  ( 9.295050272127046043, 33.31054687608394005, -9.295050272127046043 ) ) ;
#18499=DIRECTION ( 'NONE',  ( 0.000000000000000000, 1.000000000000000000, 0.000000000000000000 ) ) ;
#18504=CARTESIAN_POINT ( 'NONE',  ( 9.598844408820456309, 35.14609374999999858, -9.598844408820458085 ) ) ;
#18505=CARTESIAN_POINT ( 'NONE',  ( -13.14518615778179544, 34.40195312608393152, 0.000000000000000000 ) ) ;
#18507=CARTESIAN_POINT ( 'NONE',  ( 5.444914386472302859, 35.24531250108393010, 13.14518615778179189 ) ) ;
#18508=CARTESIAN_POINT ( 'NONE',  ( 5.622872871577878406, 35.79101562716787299, 13.57481594606304576 ) ) ;
#18529=VERTEX_POINT ( 'NONE', #19829 ) ;
#18532=CARTESIAN_POINT ( 'NONE',  ( -5.444914386472297529, 31.87187500108393223, -13.14518615778179900 ) ) ;
#18535=CARTESIAN_POINT ( 'NONE',  ( 9.598844408820459861, 35.84062500216786873, 9.598844408820456309 ) ) ;
#18566=CARTESIAN_POINT ( 'NONE',  ( 9.295050272127046043, 35.49335937608393010, -9.295050272127046043 ) ) ;
#18588=CARTESIAN_POINT ( 'NONE',  ( -13.57481594606304398, 33.11210937499999574, 5.622872871577880183 ) ) ;
#18604=DIRECTION ( 'NONE',  ( 0.000000000000000000, 1.000000000000000000, 0.000000000000000000 ) ) ;
#18608=CARTESIAN_POINT ( 'NONE',  ( 2.493653234604083739E-15, 35.74140625216787015, 13.57481594606304576 ) ) ;
#18610=AXIS2_PLACEMENT_3D ( 'NONE', #13750, #2804, #22475 ) ;
#18613=CARTESIAN_POINT ( 'NONE',  ( -13.14518615778179189, 40.00781250108393294, 5.444914386472304635 ) ) ;
#18616=CARTESIAN_POINT ( 'NONE',  ( 0.000000000000000000, 21.95886589889650509, 0.000000000000000000 ) ) ;
#18631=CARTESIAN_POINT ( 'NONE',  ( -5.444914386472297529, 32.66562500108393863, -13.14518615778179722 ) ) ;
#18634=CARTESIAN_POINT ( 'NONE',  ( -5.622872871577873966, 33.70742187499999432, -13.57481594606304753 ) ) ;
#18642=CARTESIAN_POINT ( 'NONE',  ( 9.598844408820456309, 34.35234374999999574, -9.598844408820458085 ) ) ;
#18644=CARTESIAN_POINT ( 'NONE',  ( -9.078091922698781957, 36.00000000000000711, -9.794392408849049048 ) ) ;
#18645=CARTESIAN_POINT ( 'NONE',  ( -5.622872871577873077, 40.35507812499998437, 13.57481594606304753 ) ) ;
#18647=CARTESIAN_POINT ( 'NONE',  ( -9.295050272127044266, 35.89023437608393152, 9.295050272127047819 ) ) ;
#18648=CARTESIAN_POINT ( 'NONE',  ( 5.622872871577878406, 34.20351562716788862, 13.57481594606304576 ) ) ;
#18653=CARTESIAN_POINT ( 'NONE',  ( 2.493653234604083739E-15, 34.94765625216787441, 13.57481594606304576 ) ) ;
#18654=ORIENTED_EDGE ( 'NONE', *, *, #12876, .T. ) ;
#18700=CARTESIAN_POINT ( 'NONE',  ( 2.414731522848535132E-15, 32.02070312608393010, 13.14518615778179544 ) ) ;
#18706=DIRECTION ( 'NONE',  ( 0.000000000000000000, -0.8660254037844380415, 0.5000000000000009992 ) ) ;
#18713=CARTESIAN_POINT ( 'NONE',  ( 13.14518615778179900, 35.34453125108392868, 5.444914386472293977 ) ) ;
#18745=CARTESIAN_POINT ( 'NONE',  ( 13.57481594606304753, 33.60820312716787583, -5.622872871577873966 ) ) ;
#18749=CARTESIAN_POINT ( 'NONE',  ( 2.414731522848535132E-15, 39.36289062608393152, 13.14518615778179544 ) ) ;
#18769=CYLINDRICAL_SURFACE ( 'NONE', #14941, 13.57481594606304576 ) ;
#18779=CARTESIAN_POINT ( 'NONE',  ( -13.57481594606304576, 40.20624999999999005, 0.000000000000000000 ) ) ;
#18780=CARTESIAN_POINT ( 'NONE',  ( 5.444914386472302859, 32.07031250108393294, 13.14518615778179189 ) ) ;
#18781=CARTESIAN_POINT ( 'NONE',  ( -9.598844408820458085, 33.85625000216787583, -9.598844408820458085 ) ) ;
#18791=ORIENTED_EDGE ( 'NONE', *, *, #4266, .T. ) ;
#18797=CARTESIAN_POINT ( 'NONE',  ( 0.000000000000000000, 21.36169591142201440, 23.85284712729792389 ) ) ;
#18803=CARTESIAN_POINT ( 'NONE',  ( 13.14518615778179900, 34.05468750108394005, -5.444914386472297529 ) ) ;
#18821=CARTESIAN_POINT ( 'NONE',  ( 1.137167824541903460, 36.00000000000000000, 13.09590655363594180 ) ) ;
#18833=CARTESIAN_POINT ( 'NONE',  ( -9.295050272127046043, 33.31054687608393294, -9.295050272127046043 ) ) ;
#18846=CARTESIAN_POINT ( 'NONE',  ( -13.14518615778179189, 34.25312500108393010, 5.444914386472304635 ) ) ;
#18851=FACE_OUTER_BOUND ( 'NONE', #23730, .T. ) ;
#18873=CARTESIAN_POINT ( 'NONE',  ( 13.57481594606304931, 33.50898437716787015, 5.622872871577868636 ) ) ;
#18883=EDGE_CURVE ( 'NONE', #21904, #3329, #13891, .T. ) ;
#18911=CARTESIAN_POINT ( 'NONE',  ( 13.57481594606304576, 39.01562500000000000, -1.662435489736055892E-15 ) ) ;
#18914=CARTESIAN_POINT ( 'NONE',  ( 5.622872871577871301, 32.11992187716787583, -13.57481594606304753 ) ) ;
#18936=CARTESIAN_POINT ( 'NONE',  ( 2.414731522848535132E-15, 34.60039062608393579, 13.14518615778179544 ) ) ;
#18944=AXIS2_PLACEMENT_3D ( 'NONE', #2898, #9168, #17860 ) ;
#18954=CARTESIAN_POINT ( 'NONE',  ( -7.778504368121306634, 36.00000000000000000, 10.60546543669474318 ) ) ;
#18960=CARTESIAN_POINT ( 'NONE',  ( -13.57481594606304576, 31.57421875216786944, 0.000000000000000000 ) ) ;
#18965=CARTESIAN_POINT ( 'NONE',  ( 2.493653234604083739E-15, 32.46718749999999432, 13.57481594606304576 ) ) ;
#18969=CARTESIAN_POINT ( 'NONE',  ( 9.295050272127046043, 33.90585937608393152, -9.295050272127046043 ) ) ;
#18984=CARTESIAN_POINT ( 'NONE',  ( -13.14518615778179900, 32.56640625108394005, -5.444914386472297529 ) ) ;
#19048=CARTESIAN_POINT ( 'NONE',  ( -5.444914386472299306, 32.16953125108393152, 13.14518615778179722 ) ) ;
#19049=CARTESIAN_POINT ( 'NONE',  ( -13.14518615778179722, 33.36015625108393579, -5.444914386472297529 ) ) ;
#19050=CARTESIAN_POINT ( 'NONE',  ( 13.57481594606304753, 32.81445312716787299, -5.622872871577873077 ) ) ;
#19062=ORIENTED_EDGE ( 'NONE', *, *, #733, .F. ) ;
#19069=LINE ( 'NONE', #18797, #16607 ) ;
#19075=EDGE_CURVE ( 'NONE', #22143, #25472, #10697, .T. ) ;
#19086=ADVANCED_FACE ( 'NONE', ( #18207 ), #10540, .T. ) ;
#19107=CARTESIAN_POINT ( 'NONE',  ( 13.57481594606304576, 32.66562499999999858, -1.662435489736055892E-15 ) ) ;
#19110=CARTESIAN_POINT ( 'NONE',  ( 2.414731522848535132E-15, 35.39414062608393863, 13.14518615778179544 ) ) ;
#19111=CARTESIAN_POINT ( 'NONE',  ( 13.14518615778179900, 33.75703125108393010, 5.444914386472293977 ) ) ;
#19133=CARTESIAN_POINT ( 'NONE',  ( 1.662435489736055892E-15, 36.00000000000000000, 13.57481594606304576 ) ) ;
#19160=LINE ( 'NONE', #27864, #4883 ) ;
#19164=FACE_OUTER_BOUND ( 'NONE', #12974, .T. ) ;
#19187=( LENGTH_UNIT ( ) NAMED_UNIT ( * ) SI_UNIT ( .MILLI., .METRE. ) );
#19190=ORIENTED_EDGE ( 'NONE', *, *, #6000, .T. ) ;
#19193=CARTESIAN_POINT ( 'NONE',  ( -5.444914386472297529, 33.26093750108393721, -13.14518615778179722 ) ) ;
#19194=CARTESIAN_POINT ( 'NONE',  ( -13.57481594606304753, 33.11210937716786873, -5.622872871577873077 ) ) ;
#19221=CARTESIAN_POINT ( 'NONE',  ( 13.57481594606304576, 35.84062499999999574, -1.662435489736055892E-15 ) ) ;
#19235=LINE ( 'NONE', #25646, #6180 ) ;
#19249=ORIENTED_EDGE ( 'NONE', *, *, #6386, .T. ) ;
#19250=CARTESIAN_POINT ( 'NONE',  ( -13.14518615778179189, 35.24531250108393721, 5.444914386472304635 ) ) ;
#19251=CARTESIAN_POINT ( 'NONE',  ( 5.444914386472297529, 39.71015625108393010, -13.14518615778179900 ) ) ;
#19264=EDGE_CURVE ( 'NONE', #3329, #11554, #19235, .T. ) ;
#19272=CARTESIAN_POINT ( 'NONE',  ( 5.444914386472302859, 32.07031250108393294, 13.14518615778179189 ) ) ;
#19284=FACE_OUTER_BOUND ( 'NONE', #4254, .T. ) ;
#19305=DIRECTION ( 'NONE',  ( 0.000000000000000000, 0.000000000000000000, -1.000000000000000000 ) ) ;
#19316=CARTESIAN_POINT ( 'NONE',  ( 0.000000000000000000, 10.00000000000000000, 0.000000000000000000 ) ) ;
#19330=CARTESIAN_POINT ( 'NONE',  ( 5.444914386472297529, 33.16171875108393152, -13.14518615778179722 ) ) ;
#19331=CARTESIAN_POINT ( 'NONE',  ( -8.049105076161786076E-16, 38.76757812608393294, -13.14518615778179544 ) ) ;
#19350=CARTESIAN_POINT ( 'NONE',  ( 12.53142549111940518, 36.00000000000000711, -5.200562670744389493 ) ) ;
#19362=CARTESIAN_POINT ( 'NONE',  ( -13.14518615778179900, 36.73359375108393010, -5.444914386472297529 ) ) ;
#19372=CARTESIAN_POINT ( 'NONE',  ( -7.068365687998217517, 35.99999999999998579, 11.09140360074136211 ) ) ;
#19382=VERTEX_POINT ( 'NONE', #6130 ) ;
#19383=CARTESIAN_POINT ( 'NONE',  ( 5.622872871577733633, 32.81445312500000000, -13.57481594606318254 ) ) ;
#19387=CARTESIAN_POINT ( 'NONE',  ( -5.444914386472297529, 38.22187500108393010, -13.14518615778179900 ) ) ;
#19397=DIRECTION ( 'NONE',  ( 0.000000000000000000, -0.8660254037844380415, 0.5000000000000009992 ) ) ;
#19405=CARTESIAN_POINT ( 'NONE',  ( -13.14518615778179900, 31.77265625108393365, -5.444914386472297529 ) ) ;
#19418=EDGE_CURVE ( 'NONE', #20971, #3596, #21110, .T. ) ;
#19428=CARTESIAN_POINT ( 'NONE',  ( -13.57481594606304398, 33.90585937499999858, 5.622872871577880183 ) ) ;
#19439=EDGE_CURVE ( 'NONE', #5426, #15410, #19941, .T. ) ;
#19447=VERTEX_POINT ( 'NONE', #15360 ) ;
#19453=TOROIDAL_SURFACE ( 'NONE', #26822, 23.26794919243112503, 1.000000000000000000 ) ;
#19462=CARTESIAN_POINT ( 'NONE',  ( -13.14518615778179544, 34.40195312608393152, 0.000000000000000000 ) ) ;
#19468=DIRECTION ( 'NONE',  ( -0.000000000000000000, -1.000000000000000000, -0.000000000000000000 ) ) ;
#19473=CARTESIAN_POINT ( 'NONE',  ( 9.295050272127046043, 38.66835937608393436, -9.295050272127046043 ) ) ;
#19504=CARTESIAN_POINT ( 'NONE',  ( 13.57481594606304753, 35.89023437499999858, -5.622872871577873077 ) ) ;
#19506=CARTESIAN_POINT ( 'NONE',  ( -9.295050272127044266, 36.08867187608393579, 9.295050272127047819 ) ) ;
#19521=AXIS2_PLACEMENT_3D ( 'NONE', #9093, #22495, #18214 ) ;
#19530=CARTESIAN_POINT ( 'NONE',  ( -5.444914386472297529, 34.25312500108393721, -13.14518615778179722 ) ) ;
#19531=CARTESIAN_POINT ( 'NONE',  ( -9.295050272127046043, 39.85898437608393152, -9.295050272127046043 ) ) ;
#19564=CARTESIAN_POINT ( 'NONE',  ( -13.14518615778179544, 40.55351562608393579, 0.000000000000000000 ) ) ;
#19612=CARTESIAN_POINT ( 'NONE',  ( -5.444914386472297529, 38.02343750108394005, -13.14518615778179900 ) ) ;
#19623=CONICAL_SURFACE ( 'NONE', #22358, 25.00000000000001066, 0.9599310885968833640 ) ;
#19631=CARTESIAN_POINT ( 'NONE',  ( 3.829562757992932998, 36.00000000000000000, 12.63428651647562795 ) ) ;
#19639=DIRECTION ( 'NONE',  ( 0.000000000000000000, 0.000000000000000000, 1.000000000000000000 ) ) ;
#19641=CARTESIAN_POINT ( 'NONE',  ( 9.598844408820456309, 38.32109374999999574, -9.598844408820458085 ) ) ;
#19643=CARTESIAN_POINT ( 'NONE',  ( 13.14518615778179544, 38.76757812608393294, -1.609821015232357215E-15 ) ) ;
#19662=ORIENTED_EDGE ( 'NONE', *, *, #3875, .T. ) ;
#19669=CARTESIAN_POINT ( 'NONE',  ( 13.14518615778179722, 35.64218750108393863, -5.444914386472297529 ) ) ;
#19671=CARTESIAN_POINT ( 'NONE',  ( 5.444914386472302859, 39.41250000108393436, 13.14518615778179189 ) ) ;
#19700=ORIENTED_EDGE ( 'NONE', *, *, #14844, .F. ) ;
#19702=CARTESIAN_POINT ( 'NONE',  ( 13.14518615778179900, 39.41250000108393436, -5.444914386472297529 ) ) ;
#19707=( BOUNDED_CURVE ( )  B_SPLINE_CURVE ( 2, ( #17926, #409, #20503, #9369, #11780, #9654, #696, #2826, #5109 ),
 .UNSPECIFIED., .F., .F. ) 
 B_SPLINE_CURVE_WITH_KNOTS ( ( 3, 2, 2, 2, 3 ),
 ( 0.5625000000000004441, 0.5729166666666669627, 0.5833333333333337034, 0.5937500000000002220, 0.6041666666666668517 ),
 .UNSPECIFIED. ) 
 CURVE ( )  GEOMETRIC_REPRESENTATION_ITEM ( )  RATIONAL_B_SPLINE_CURVE ( ( 0.9999999999999967804, 0.9238795325112899581, 1.000000000000000000, 0.9238795325112867385, 1.000000000000000000, 0.9238795325112867385, 1.000000000000000000, 0.9238795325112850731, 1.000000000000001554 ) ) 
 REPRESENTATION_ITEM ( '' )  );
#19710=CARTESIAN_POINT ( 'NONE',  ( 1.662435489736055892E-15, 31.00000000000000000, 13.57481594606304576 ) ) ;
#19744=ORIENTED_EDGE ( 'NONE', *, *, #19439, .F. ) ;
#19750=CARTESIAN_POINT ( 'NONE',  ( -13.14518615778179900, 38.91640625108393436, -5.444914386472297529 ) ) ;
#19757=CARTESIAN_POINT ( 'NONE',  ( 0.000000000000000000, 0.4999999999999970024, 0.000000000000000000 ) ) ;
#19770=CARTESIAN_POINT ( 'NONE',  ( 5.364947964715831574, 35.99999999999997158, 12.09311862596023701 ) ) ;
#19772=ADVANCED_FACE ( 'NONE', ( #23212 ), #21069, .F. ) ;
#19783=CARTESIAN_POINT ( 'NONE',  ( -13.57481594606304576, 37.08085937499999574, 5.622872871577880183 ) ) ;
#19786=CARTESIAN_POINT ( 'NONE',  ( 5.444914386472297529, 38.12265625108393152, -13.14518615778179900 ) ) ;
#19790=CYLINDRICAL_SURFACE ( 'NONE', #1499, 13.57481594606304576 ) ;
#19808=DIRECTION ( 'NONE',  ( 0.000000000000000000, 0.000000000000000000, 1.000000000000000000 ) ) ;
#19812=CARTESIAN_POINT ( 'NONE',  ( -5.444914386472299306, 32.96328125108393436, 13.14518615778179722 ) ) ;
#19813=CARTESIAN_POINT ( 'NONE',  ( -9.295050272127044266, 40.05742187608393579, 9.295050272127047819 ) ) ;
#19814=UNCERTAINTY_MEASURE_WITH_UNIT (LENGTH_MEASURE( 1.000000000000000082E-05 ), #13163, 'distance_accuracy_value', 'NONE');
#19823=CARTESIAN_POINT ( 'NONE',  ( -8.312177448680279460E-16, 34.45156249999999432, -13.57481594606304576 ) ) ;
#19828=AXIS2_PLACEMENT_3D ( 'NONE', #11345, #11628, #22637 ) ;
#19829=CARTESIAN_POINT ( 'NONE',  ( 0.000000000000000000, 1.500000000000001332, 24.13397459621556607 ) ) ;
#19837=( BOUNDED_CURVE ( )  B_SPLINE_CURVE ( 2, ( #18608, #7770, #18179, #24882, #18326, #22752, #13884, #664, #18031 ),
 .UNSPECIFIED., .F., .F. ) 
 B_SPLINE_CURVE_WITH_KNOTS ( ( 3, 2, 2, 2, 3 ),
 ( 0.4791666666666667962, 0.4895833333333333703, 0.5000000000000000000, 0.5104166666666665186, 0.5208333333333332593 ),
 .UNSPECIFIED. ) 
 CURVE ( )  GEOMETRIC_REPRESENTATION_ITEM ( )  RATIONAL_B_SPLINE_CURVE ( ( 0.9999999999999992228, 0.9238795325112875156, 1.000000000000000000, 0.9238795325112867385, 1.000000000000000000, 0.9238795325112867385, 1.000000000000000000, 0.9238795325112875156, 0.9999999999999992228 ) ) 
 REPRESENTATION_ITEM ( '' )  );
#19839=VERTEX_POINT ( 'NONE', #24041 ) ;
#19844=CARTESIAN_POINT ( 'NONE',  ( 5.444914386472297529, 38.71796875108393721, -13.14518615778179900 ) ) ;
#19845=VECTOR ( 'NONE', #24147, 1000.000000000000000 ) ;
#19854=ORIENTED_EDGE ( 'NONE', *, *, #6701, .F. ) ;
#19886=CARTESIAN_POINT ( 'NONE',  ( 0.000000000000000000, 29.95886589889650509, 11.57481594606304576 ) ) ;
#19896=CARTESIAN_POINT ( 'NONE',  ( -5.444914386472299306, 39.11484375108394573, 13.14518615778179722 ) ) ;
#19916=CARTESIAN_POINT ( 'NONE',  ( 7.754123975995396378, 35.99999999999999289, 10.77549638133713472 ) ) ;
#19927=CARTESIAN_POINT ( 'NONE',  ( -8.312177448680279460E-16, 32.16953125216787157, -13.57481594606304576 ) ) ;
#19928=CARTESIAN_POINT ( 'NONE',  ( 9.598844408820456309, 35.93984374999999432, -9.598844408820458085 ) ) ;
#19930=CARTESIAN_POINT ( 'NONE',  ( 5.444914386472302859, 37.03125000108393294, 13.14518615778179189 ) ) ;
#19932=EDGE_CURVE ( 'NONE', #21429, #12537, #25300, .T. ) ;
#19936=DIRECTION ( 'NONE',  ( -0.000000000000000000, -1.000000000000000000, -0.000000000000000000 ) ) ;
#19941=LINE ( 'NONE', #6537, #721 ) ;
#19956=ORIENTED_EDGE ( 'NONE', *, *, #19075, .F. ) ;
#19960=CARTESIAN_POINT ( 'NONE',  ( -9.295050272127046043, 36.68398437608393436, -9.295050272127046043 ) ) ;
#19989=VERTEX_POINT ( 'NONE', #20189 ) ;
#19994=CARTESIAN_POINT ( 'NONE',  ( -9.295050272127044266, 39.85898437608393152, 9.295050272127047819 ) ) ;
#20013=ORIENTED_EDGE ( 'NONE', *, *, #5180, .F. ) ;
#20027=ORIENTED_EDGE ( 'NONE', *, *, #16815, .T. ) ;
#20043=CARTESIAN_POINT ( 'NONE',  ( -13.14518615778179189, 35.84062500108394289, 5.444914386472304635 ) ) ;
#20068=CARTESIAN_POINT ( 'NONE',  ( -9.598844408820458085, 40.20625000216787726, -9.598844408820458085 ) ) ;
#20075=CARTESIAN_POINT ( 'NONE',  ( -8.312177448680279460E-16, 36.03906250000000000, -13.57481594606304576 ) ) ;
#20076=APPLICATION_CONTEXT ( 'automotive_design' ) ;
#20078=CARTESIAN_POINT ( 'NONE',  ( 2.414731522848535132E-15, 33.01289062608393721, 13.14518615778179544 ) ) ;
#20082=CARTESIAN_POINT ( 'NONE',  ( -9.598844408820458085, 36.23750000216787726, -9.598844408820458085 ) ) ;
#20094=CARTESIAN_POINT ( 'NONE',  ( 2.493653234604083739E-15, 34.84843749999999574, 13.57481594606304576 ) ) ;
#20106=CARTESIAN_POINT ( 'NONE',  ( 13.14518615778179900, 35.54296875108394715, 5.444914386472293977 ) ) ;
#20136=CARTESIAN_POINT ( 'NONE',  ( -5.444914386472297529, 37.22968750108393721, -13.14518615778179900 ) ) ;
#20183=CARTESIAN_POINT ( 'NONE',  ( 13.14518615778179900, 35.44375000108393436, -5.444914386472297529 ) ) ;
#20189=CARTESIAN_POINT ( 'NONE',  ( 2.493653234604083739E-15, 34.05468749999999289, 13.57481594606304576 ) ) ;
#20203=CARTESIAN_POINT ( 'NONE',  ( 13.57481594606304931, 38.27148437716787299, 5.622872871577869525 ) ) ;
#20206=CARTESIAN_POINT ( 'NONE',  ( -5.622872871577965448, 33.31054687716787299, 13.57481594606295161 ) ) ;
#20207=DIRECTION ( 'NONE',  ( -0.000000000000000000, -1.000000000000000000, -0.000000000000000000 ) ) ;
#20209=EDGE_LOOP ( 'NONE', ( #7, #20013, #6307, #148 ) ) ;
#20210=FACE_OUTER_BOUND ( 'NONE', #26858, .T. ) ;
#20212=CARTESIAN_POINT ( 'NONE',  ( 13.57481594606304931, 34.20351562499999432, 5.622872871577869525 ) ) ;
#20215=CARTESIAN_POINT ( 'NONE',  ( 5.444914386472302859, 33.85625000108393579, 13.14518615778179189 ) ) ;
#20217=CARTESIAN_POINT ( 'NONE',  ( -13.14518615778179189, 35.84062500108394289, 5.444914386472304635 ) ) ;
#20218=CARTESIAN_POINT ( 'NONE',  ( 2.493653234604083739E-15, 34.94765625216787441, 13.57481594606304576 ) ) ;
#20242=CARTESIAN_POINT ( 'NONE',  ( 5.444914386472302859, 35.44375000108393436, 13.14518615778179189 ) ) ;
#20264=CARTESIAN_POINT ( 'NONE',  ( 0.000000000000000000, 1.000000000000000000, 23.26794919243112503 ) ) ;
#20273=CARTESIAN_POINT ( 'NONE',  ( 13.14518615778179900, 37.82500000108392868, -5.444914386472297529 ) ) ;
#20283=ORIENTED_EDGE ( 'NONE', *, *, #20675, .F. ) ;
#20304=VERTEX_POINT ( 'NONE', #21032 ) ;
#20306=ADVANCED_FACE ( 'NONE', ( #19164 ), #12539, .T. ) ;
#20315=CARTESIAN_POINT ( 'NONE',  ( -9.598844408820458085, 33.85625000216787583, -9.598844408820458085 ) ) ;
#20325=CARTESIAN_POINT ( 'NONE',  ( 9.295050272127046043, 36.28710937608393294, -9.295050272127046043 ) ) ;
#20326=LINE ( 'NONE', #11603, #16523 ) ;
#20337=EDGE_CURVE ( 'NONE', #25472, #22143, #13911, .T. ) ;
#20348=AXIS2_PLACEMENT_3D ( 'NONE', #14128, #22027, #20711 ) ;
#20349=CARTESIAN_POINT ( 'NONE',  ( -9.295050272127046043, 31.92148437608393508, -9.295050272127046043 ) ) ;
#20352=CARTESIAN_POINT ( 'NONE',  ( 5.622872871577878406, 38.96601562716787015, 13.57481594606304576 ) ) ;
#20359=CARTESIAN_POINT ( 'NONE',  ( 13.57481594606304931, 32.61601562499999574, 5.622872871577869525 ) ) ;
#20362=CARTESIAN_POINT ( 'NONE',  ( 13.14518615778179900, 33.95546875108393436, 5.444914386472293977 ) ) ;
#20366=CARTESIAN_POINT ( 'NONE',  ( 13.57481594606304753, 35.19570312716788152, -5.622872871577873077 ) ) ;
#20376=EDGE_LOOP ( 'NONE', ( #26405, #1867, #16008, #16961 ) ) ;
#20389=CARTESIAN_POINT ( 'NONE',  ( 9.295050272127047819, 37.87460937608393863, 9.295050272127046043 ) ) ;
#20415=ORIENTED_EDGE ( 'NONE', *, *, #19264, .T. ) ;
#20422=CARTESIAN_POINT ( 'NONE',  ( -8.049105076161786076E-16, 35.59257812608393579, -13.14518615778179544 ) ) ;
#20429=CARTESIAN_POINT ( 'NONE',  ( -13.14518615778179189, 36.03906250108394005, 5.444914386472304635 ) ) ;
#20433=ORIENTED_EDGE ( 'NONE', *, *, #451, .T. ) ;
#20448=ORIENTED_EDGE ( 'NONE', *, *, #13672, .T. ) ;
#20463=CARTESIAN_POINT ( 'NONE',  ( 2.493653234604083739E-15, 34.15390625216787157, 13.57481594606304576 ) ) ;
#20468=STYLED_ITEM ( 'NONE', ( #2376 ), #11047 ) ;
#20494=CARTESIAN_POINT ( 'NONE',  ( -13.14518615778179189, 33.65781250108393152, 5.444914386472304635 ) ) ;
#20497=CARTESIAN_POINT ( 'NONE',  ( 13.57481594606304576, 39.90859375216787441, -1.662435489736055892E-15 ) ) ;
#20503=CARTESIAN_POINT ( 'NONE',  ( -9.598844408820454532, 35.54296874999999289, 9.598844408820459861 ) ) ;
#20505=CARTESIAN_POINT ( 'NONE',  ( -9.598844408820458085, 32.96328124999999432, -9.598844408820458085 ) ) ;
#20507=CARTESIAN_POINT ( 'NONE',  ( -13.14518615778179544, 35.19570312608393436, 0.000000000000000000 ) ) ;
#20509=CARTESIAN_POINT ( 'NONE',  ( -13.14518615778179544, 34.99726562608393721, 0.000000000000000000 ) ) ;
#20511=CARTESIAN_POINT ( 'NONE',  ( -13.57481594606304576, 37.13046875216787868, 0.000000000000000000 ) ) ;
#20535=ORIENTED_EDGE ( 'NONE', *, *, #13284, .T. ) ;
#20536=CARTESIAN_POINT ( 'NONE',  ( -5.444914386472299306, 37.72578125108395142, 13.14518615778179722 ) ) ;
#20568=CARTESIAN_POINT ( 'NONE',  ( -9.295050272127046043, 38.07304687608393579, -9.295050272127046043 ) ) ;
#20594=DIRECTION ( 'NONE',  ( 6.123233995736778362E-17, 0.8660254037844380415, -0.5000000000000009992 ) ) ;
#20601=( BOUNDED_CURVE ( )  B_SPLINE_CURVE ( 2, ( #20463, #24590, #658, #16020, #13735, #9330, #20315, #18025, #22459 ),
 .UNSPECIFIED., .F., .F. ) 
 B_SPLINE_CURVE_WITH_KNOTS ( ( 3, 2, 2, 2, 3 ),
 ( 0.6458333333333333703, 0.6562500000000000000, 0.6666666666666665186, 0.6770833333333332593, 0.6874999999999997780 ),
 .UNSPECIFIED. ) 
 CURVE ( )  GEOMETRIC_REPRESENTATION_ITEM ( )  RATIONAL_B_SPLINE_CURVE ( ( 1.000000000000000000, 0.9238795325112867385, 1.000000000000000000, 0.9238795325112867385, 1.000000000000000000, 0.9238795325112867385, 1.000000000000000000, 0.9238795325112884038, 0.9999999999999983347 ) ) 
 REPRESENTATION_ITEM ( '' )  );
#20605=ORIENTED_EDGE ( 'NONE', *, *, #11904, .T. ) ;
#20611=FACE_OUTER_BOUND ( 'NONE', #21469, .T. ) ;
#20620=VECTOR ( 'NONE', #18172, 1000.000000000000000 ) ;
#20623=EDGE_CURVE ( 'NONE', #12114, #13023, #15433, .T. ) ;
#20633=CARTESIAN_POINT ( 'NONE',  ( 13.14518615778179722, 33.16171875108393863, 5.444914386472293977 ) ) ;
#20636=CARTESIAN_POINT ( 'NONE',  ( -13.57481594606304576, 37.92421875216787441, 0.000000000000000000 ) ) ;
#20638=FACE_OUTER_BOUND ( 'NONE', #27644, .T. ) ;
#20645=CARTESIAN_POINT ( 'NONE',  ( -13.57481594606304576, 35.44374999999999432, 0.000000000000000000 ) ) ;
#20646=CARTESIAN_POINT ( 'NONE',  ( -8.669112105337029917, 36.00000000000002842, -10.16963847934323262 ) ) ;
#20647=CARTESIAN_POINT ( 'NONE',  ( -9.295050272127044266, 33.70742187608393436, 9.295050272127047819 ) ) ;
#20650=CARTESIAN_POINT ( 'NONE',  ( -5.622872871577873077, 35.69179687716786731, 13.57481594606304753 ) ) ;
#20654=LINE ( 'NONE', #22935, #27603 ) ;
#20664=DIRECTION ( 'NONE',  ( 0.000000000000000000, 0.000000000000000000, 1.000000000000000000 ) ) ;
#20675=EDGE_CURVE ( 'NONE', #17432, #19989, #1827, .T. ) ;
#20677=CARTESIAN_POINT ( 'NONE',  ( 5.444914386472302859, 32.26875000108393721, 13.14518615778179189 ) ) ;
#20709=CARTESIAN_POINT ( 'NONE',  ( -13.14518615778179189, 36.63437500108393152, 5.444914386472304635 ) ) ;
#20711=DIRECTION ( 'NONE',  ( 0.000000000000000000, 0.000000000000000000, 1.000000000000000000 ) ) ;
#20753=CARTESIAN_POINT ( 'NONE',  ( -13.14518615778179900, 40.70234375108393721, -5.444914386472297529 ) ) ;
#20769=CARTESIAN_POINT ( 'NONE',  ( -13.14518615778179722, 31.97109375108393792, -5.444914386472297529 ) ) ;
#20782=CARTESIAN_POINT ( 'NONE',  ( -9.598844408820454532, 33.16171874999999858, 9.598844408820459861 ) ) ;
#20785=CARTESIAN_POINT ( 'NONE',  ( -5.444914386472297529, 32.66562500108393863, -13.14518615778179900 ) ) ;
#20788=CARTESIAN_POINT ( 'NONE',  ( -13.57481594606304576, 34.00507812716787015, 5.622872871577880183 ) ) ;
#20799=ORIENTED_EDGE ( 'NONE', *, *, #17684, .F. ) ;
#20810=CARTESIAN_POINT ( 'NONE',  ( -13.14518615778179900, 32.76484375108393010, -5.444914386472297529 ) ) ;
#20813=EDGE_CURVE ( 'NONE', #25968, #6997, #3071, .T. ) ;
#20846=CARTESIAN_POINT ( 'NONE',  ( 9.295050272127047819, 32.11992187608393579, 9.295050272127046043 ) ) ;
#20858=CARTESIAN_POINT ( 'NONE',  ( 5.444914386472297529, 36.33671875108394289, -13.14518615778179900 ) ) ;
#20873=CARTESIAN_POINT ( 'NONE',  ( -2.743444426250911979E-15, 0.4999999999999970024, -22.40192378864669465 ) ) ;
#20882=CARTESIAN_POINT ( 'NONE',  ( 0.000000000000000000, 0.000000000000000000, 0.000000000000000000 ) ) ;
#20890=CIRCLE ( 'NONE', #12664, 11.57481594606304576 ) ;
#20893=CARTESIAN_POINT ( 'NONE',  ( 13.14518615778179900, 39.61093750108393863, -5.444914386472297529 ) ) ;
#20896=DIRECTION ( 'NONE',  ( 0.000000000000000000, 1.000000000000000000, 0.000000000000000000 ) ) ;
#20899=ORIENTED_EDGE ( 'NONE', *, *, #3086, .F. ) ;
#20902=PRODUCT_DEFINITION_CONTEXT ( 'detailed design', #3147, 'design' ) ;
#20925=CARTESIAN_POINT ( 'NONE',  ( -5.622872871577873077, 39.26367187499999289, -13.57481594606304753 ) ) ;
#20926=CARTESIAN_POINT ( 'NONE',  ( 6.944423797152706079, 31.55306878032414986, -11.16113333171310451 ) ) ;
#20927=CARTESIAN_POINT ( 'NONE',  ( 9.598844408820459861, 31.87187500216787228, 9.598844408820456309 ) ) ;
#20950=CARTESIAN_POINT ( 'NONE',  ( 9.295050272127046043, 34.10429687608393579, -9.295050272127046043 ) ) ;
#20971=VERTEX_POINT ( 'NONE', #4174 ) ;
#20975=CARTESIAN_POINT ( 'NONE',  ( -13.57481594606304398, 31.62382812716787228, 5.622872871577880183 ) ) ;
#20983=CARTESIAN_POINT ( 'NONE',  ( 9.295050272127046043, 34.69960937608393436, -9.295050272127046043 ) ) ;
#20997=CARTESIAN_POINT ( 'NONE',  ( 5.444914386472302859, 36.03906250108394005, 13.14518615778179189 ) ) ;
#21016=DIRECTION ( 'NONE',  ( 0.000000000000000000, 1.000000000000000000, 0.000000000000000000 ) ) ;
#21019=ADVANCED_FACE ( 'NONE', ( #5696 ), #285, .T. ) ;
#21032=CARTESIAN_POINT ( 'NONE',  ( -8.312177448680279460E-16, 32.86406249999999574, -13.57481594606304576 ) ) ;
#21043=EDGE_CURVE ( 'NONE', #15854, #15131, #22662, .T. ) ;
#21058=CARTESIAN_POINT ( 'NONE',  ( 2.493653234604083739E-15, 32.46718749999999432, 13.57481594606304576 ) ) ;
#21060=CARTESIAN_POINT ( 'NONE',  ( 13.57481594606304931, 40.55351562499998863, 5.622872871577869525 ) ) ;
#21061=CARTESIAN_POINT ( 'NONE',  ( 2.414731522848535132E-15, 32.81445312608393294, 13.14518615778179544 ) ) ;
#21063=CARTESIAN_POINT ( 'NONE',  ( 2.493653234604083739E-15, 32.56640625216787299, 13.57481594606304576 ) ) ;
#21068=CARTESIAN_POINT ( 'NONE',  ( 13.57481594606304753, 35.19570312716787441, -5.622872871577873966 ) ) ;
#21069=CYLINDRICAL_SURFACE ( 'NONE', #26220, 11.57481594606304576 ) ;
#21085=CARTESIAN_POINT ( 'NONE',  ( 9.295050272127046043, 32.51679687608393721, -9.295050272127046043 ) ) ;
#21090=EDGE_CURVE ( 'NONE', #10399, #21990, #16080, .T. ) ;
#21103=CARTESIAN_POINT ( 'NONE',  ( -9.713547494048821562, 36.00000000000000000, 8.898183052316806396 ) ) ;
#21110=B_SPLINE_CURVE_WITH_KNOTS ( 'NONE', 3,
 ( #3583, #27528, #6264, #16945, #10107, #1864, #8395, #5995, #1591, #21103, #10664, #14937, #18954, #19372, #23659, #21518, #1997, #28076, #17226, #27662, #8124, #5726, #23109, #16820, #18821 ),
 .UNSPECIFIED., .F., .F.,
 ( 4, 2, 2, 2, 2, 2, 2, 1, 2, 2, 2, 2, 4 ),
 ( 0.000000000000000000, 0.001301161269048867718, 0.002602322538097735435, 0.005204645076195470003, 0.007806967614293204571, 0.01040929015239093480, 0.01171045142143979818, 0.01301161269048865983, 0.01431277395953752495, 0.01561393522858638833, 0.01821625776668411162, 0.01951741903573297673, 0.02081858030478183838 ),
 .UNSPECIFIED. ) ;
#21116=CARTESIAN_POINT ( 'NONE',  ( 13.14518615778179900, 34.55078125108393294, 5.444914386472293977 ) ) ;
#21132=CARTESIAN_POINT ( 'NONE',  ( -13.14518615778179900, 33.36015625108393579, -5.444914386472297529 ) ) ;
#21161=CARTESIAN_POINT ( 'NONE',  ( 13.57481594606304576, 33.55859375216787299, -1.662435489736055892E-15 ) ) ;
#21163=DIRECTION ( 'NONE',  ( -0.000000000000000000, -1.000000000000000000, -0.000000000000000000 ) ) ;
#21198=CARTESIAN_POINT ( 'NONE',  ( 5.444914386472302859, 32.26875000108393721, 13.14518615778179189 ) ) ;
#21199=CARTESIAN_POINT ( 'NONE',  ( -13.14518615778179544, 33.40976562608393863, 0.000000000000000000 ) ) ;
#21201=CARTESIAN_POINT ( 'NONE',  ( -9.598844408820454532, 32.46718750216787441, 9.598844408820459861 ) ) ;
#21208=CARTESIAN_POINT ( 'NONE',  ( 2.493653234604083739E-15, 34.15390625216787157, 13.57481594606304576 ) ) ;
#21235=PRODUCT_CONTEXT ( 'NONE', #20076, 'mechanical' ) ;
#21254=CARTESIAN_POINT ( 'NONE',  ( 5.622872871577786924, 32.51679687499999716, 13.57481594606313813 ) ) ;
#21258=CARTESIAN_POINT ( 'NONE',  ( 2.414731522848535132E-15, 32.81445312608393294, 13.14518615778179544 ) ) ;
#21273=CARTESIAN_POINT ( 'NONE',  ( 5.444914386472297529, 32.36796875108393579, -13.14518615778179900 ) ) ;
#21286=CARTESIAN_POINT ( 'NONE',  ( 0.000000000000000000, 1.000000000000000000, 0.000000000000000000 ) ) ;
#21302=CARTESIAN_POINT ( 'NONE',  ( -2.921131288499653970E-15, 21.36169591142201440, -23.85284712729792389 ) ) ;
#21325=DIRECTION ( 'NONE',  ( 0.000000000000000000, 0.8660254037844380415, 0.5000000000000009992 ) ) ;
#21340=CARTESIAN_POINT ( 'NONE',  ( 3.755638155860017591, 31.78804748261757140, -13.14518615778179367 ) ) ;
#21342=CARTESIAN_POINT ( 'NONE',  ( -9.598844408820454532, 34.05468750216788010, 9.598844408820459861 ) ) ;
#21375=DIRECTION ( 'NONE',  ( -0.000000000000000000, -1.000000000000000000, -0.000000000000000000 ) ) ;
#21392=CARTESIAN_POINT ( 'NONE',  ( -13.57481594606304753, 31.52460937716787370, -5.622872871577872189 ) ) ;
#21402=CARTESIAN_POINT ( 'NONE',  ( -13.09590655363597733, 35.99999999999999289, 1.137167824541468031 ) ) ;
#21403=CARTESIAN_POINT ( 'NONE',  ( 5.444914386472302859, 34.45156250108393436, 13.14518615778179189 ) ) ;
#21419=CARTESIAN_POINT ( 'NONE',  ( 13.14518615778179900, 33.06250000108393294, -5.444914386472297529 ) ) ;
#21429=VERTEX_POINT ( 'NONE', #20873 ) ;
#21435=CARTESIAN_POINT ( 'NONE',  ( 0.000000000000000000, 0.000000000000000000, 23.26794919243112858 ) ) ;
#21444=ORIENTED_EDGE ( 'NONE', *, *, #28153, .T. ) ;
#21450=CIRCLE ( 'NONE', #10504, 25.00000000000001066 ) ;
#21469=EDGE_LOOP ( 'NONE', ( #19854, #18791, #4778, #13587 ) ) ;
#21477=CARTESIAN_POINT ( 'NONE',  ( 9.295050272127047819, 32.91367187608393152, 9.295050272127046043 ) ) ;
#21478=CARTESIAN_POINT ( 'NONE',  ( -5.444914386472297529, 39.61093750108393152, -13.14518615778179900 ) ) ;
#21502=CARTESIAN_POINT ( 'NONE',  ( 9.598844408820459861, 35.74140624999999716, 9.598844408820456309 ) ) ;
#21507=CARTESIAN_POINT ( 'NONE',  ( 13.14518615778179900, 37.13046875108393863, 5.444914386472293977 ) ) ;
#21518=CARTESIAN_POINT ( 'NONE',  ( -5.569058551902509535, 36.00000000000000000, 11.91493531101285619 ) ) ;
#21531=CARTESIAN_POINT ( 'NONE',  ( -8.312177448680279460E-16, 32.86406249999999574, -13.57481594606304576 ) ) ;
#21534=CARTESIAN_POINT ( 'NONE',  ( -13.14518615778179544, 35.99464330212367003, 0.5696516875508460531 ) ) ;
#21535=CARTESIAN_POINT ( 'NONE',  ( 2.414731522848535132E-15, 38.56914062608393579, 13.14518615778179544 ) ) ;
#21556=CARTESIAN_POINT ( 'NONE',  ( -9.295050272127046043, 34.10429687608393579, -9.295050272127046043 ) ) ;
#21573=CARTESIAN_POINT ( 'NONE',  ( 9.295050272127047819, 40.05742187608392868, 9.295050272127046043 ) ) ;
#21604=CARTESIAN_POINT ( 'NONE',  ( 5.444914386472302859, 33.85625000108393579, 13.14518615778179189 ) ) ;
#21614=ORIENTED_EDGE ( 'NONE', *, *, #12329, .F. ) ;
#21618=CARTESIAN_POINT ( 'NONE',  ( -8.049105076161786076E-16, 37.97382812608393721, -13.14518615778179544 ) ) ;
#21639=CARTESIAN_POINT ( 'NONE',  ( 13.45411265623090280, 36.00000000000000000, 0.6772748633549623420 ) ) ;
#21650=CARTESIAN_POINT ( 'NONE',  ( 13.57481594606304753, 36.68398437499999432, -5.622872871577873077 ) ) ;
#21652=CARTESIAN_POINT ( 'NONE',  ( -5.444914386472299306, 36.13828125108393863, 13.14518615778179722 ) ) ;
#21678=CARTESIAN_POINT ( 'NONE',  ( -13.14518615778179722, 34.35234375108393579, -5.444914386472297529 ) ) ;
#21680=CARTESIAN_POINT ( 'NONE',  ( -8.049105076161786076E-16, 38.96601562608393721, -13.14518615778179544 ) ) ;
#21689=VECTOR ( 'NONE', #24653, 1000.000000000000000 ) ;
#21716=CARTESIAN_POINT ( 'NONE',  ( -13.14518615778179189, 38.22187500108393010, 5.444914386472304635 ) ) ;
#21718=EDGE_CURVE ( 'NONE', #18166, #25525, #17130, .T. ) ;
#21764=CARTESIAN_POINT ( 'NONE',  ( 13.14518615778179544, 40.15664062608393436, -1.609821015232357215E-15 ) ) ;
#21781=CARTESIAN_POINT ( 'NONE',  ( 12.07727640983550188, 36.00000000000000000, -6.197985357349471869 ) ) ;
#21792=CARTESIAN_POINT ( 'NONE',  ( 13.57481594606304931, 37.37851562499999858, 5.622872871577869525 ) ) ;
#21794=CARTESIAN_POINT ( 'NONE',  ( 4.157286354961724939, 36.00000000000000000, -12.92256159328856135 ) ) ;
#21795=CARTESIAN_POINT ( 'NONE',  ( -13.14518615778179189, 38.42031250108393436, 5.444914386472304635 ) ) ;
#21820=CARTESIAN_POINT ( 'NONE',  ( 0.000000000000000000, 1.000000000000000000, 0.000000000000000000 ) ) ;
#21823=CARTESIAN_POINT ( 'NONE',  ( -13.14518615778179189, 34.45156250108394147, 5.444914386472304635 ) ) ;
#21824=CARTESIAN_POINT ( 'NONE',  ( -13.14518615778179544, 39.16445312608393436, 0.000000000000000000 ) ) ;
#21837=CARTESIAN_POINT ( 'NONE',  ( 0.000000000000000000, 0.000000000000000000, 0.000000000000000000 ) ) ;
#21847=DIRECTION ( 'NONE',  ( -0.000000000000000000, -1.000000000000000000, -0.000000000000000000 ) ) ;
#21882=VECTOR ( 'NONE', #6490, 1000.000000000000000 ) ;
#21885=( BOUNDED_SURFACE ( )  B_SPLINE_SURFACE ( 1, 2, ( 
 ( #19564, #48, #10851, #6871, #2612, #13407, #11274, #17562, #17709, #2190, #21573, #26552, #2332, #15556, #19994, #4322, #13120, #15267, #9017, #17421, #23986, #14990, #10990, #19702, #28125, #24265, #4601, #2048, #26266, #21992, #26412, #474, #23707, #26120, #6726, #25982, #15412, #19844, #24128, #13260, #4747, #331, #10716, #17279, #6452, #15123, #12980, #21716, #18131, #15703, #20568, #14126, #22705, #7292, #13977, #20273, #24695, #2754, #5457, #13555, #3173, #5173, #9432, #7007, #11845, #13836, #7580, #20136, #9720, #26697, #17988, #26987, #22562, #26843, #2885, #24550, #11985, #7432, #9291, #20709, #22847, #22416, #9577, #16274, #3314, #5033, #15981, #615, #24972, #7147, #18422, #3028, #11697, #1048, #16127, #27130, #24404, #4892, #1191, #9859, #20422, #906, #18566, #18281, #22279, #24834, #11417, #15841, #13699, #11556, #5316, #758, #3598, #1464, #10120, #5876, #9991, #27268, #20983, #12119, #4011, #21116, #23535, #21403, #12395, #14546, #27677, #1603, #23261, #14674, #1881, #6010, #25249, #10544, #18969, #7724, #3735, #19111, #16416, #10259, #12256, #8140, #16834, #14810, #16558, #1739, #18833, #10405, #25113, #27540, #27819, #12677, #3868, #12530, #7997, #8272, #21258, #7864, #25530, #22986, #23395, #5600, #5739, #16963, #16696, #25663, #6145, #3454, #25395, #14266, #20846, #1324, #18700, #14406, #27403, #23123, #12812, #4568, #4287, #10816, #6689, #25946, #8410 ),
 ( #22104, #23809, #12944, #15090, #11101, #26379, #17671, #6835, #4433, #21961, #6421, #25802, #2582, #6553, #19813, #15525, #28092, #17388, #19531, #13085, #8555, #19251, #27953, #26086, #8981, #2300, #17244, #19671, #2440, #13, #10960, #13229, #21824, #8697, #297, #15378, #21680, #24233, #15233, #4714, #154, #2011, #23951, #13374, #21535, #8839, #17529, #2154, #10680, #4152, #17099, #19387, #26231, #6279, #24093, #14955, #23675, #1019, #20389, #9690, #7113, #20536, #24941, #18389, #5427, #15813, #15672, #9547, #11384, #13805, #9399, #2856, #4859, #24664, #26957, #2995, #22245, #876, #2723, #6976, #5005, #22815, #19960, #11814, #27095, #18098, #7400, #727, #26667, #14096, #24518, #13668, #22382, #3146, #7548, #16244, #11242, #5139, #13947, #11523, #17816, #437, #26811, #9123, #26520, #20106, #7259, #20242, #22528, #584, #24371, #13525, #15949, #9262, #11668, #17956, #18249, #22674, #16093, #24801, #5283, #25362, #12222, #3835, #18936, #16526, #10751, #27509, #19462, #5842, #14235, #10090, #16800, #25083, #20950, #18803, #25218, #5571, #16384, #21604, #22957, #14511, #26014, #3419, #11954, #1431, #2082, #12366, #28159, #27373, #12874, #17315, #8626, #6485, #7832, #7693, #1573, #12087, #23228, #7965, #23089, #20810, #16666, #27645, #3705, #1290, #21085, #9959, #27237, #5708, #15159, #20677, #3283, #1160, #14374, #14644, #9825, #3563, #23363, #18532, #8106, #25497, #10226 ) ),
 .UNSPECIFIED., .F., .F., .F. ) 
 B_SPLINE_SURFACE_WITH_KNOTS ( ( 2, 2 ),
 ( 3, 2, 2, 2, 2, 2, 2, 2, 2, 2, 2, 2, 2, 2, 2, 2, 2, 2, 2, 2, 2, 2, 2, 2, 2, 2, 2, 2, 2, 2, 2, 2, 2, 2, 2, 2, 2, 2, 2, 2, 2, 2, 2, 2, 2, 2, 2, 2, 2, 2, 2, 2, 2, 2, 2, 2, 2, 2, 2, 2, 2, 2, 2, 2, 2, 2, 2, 2, 2, 2, 2, 2, 2, 2, 2, 2, 2, 2, 2, 2, 2, 2, 2, 2, 2, 2, 2, 2, 2, 2, 2, 3 ),
 ( 0.000000000000000000, 1.000000000000000000 ),
 ( 0.000000000000000000, 0.01041666666666666609, 0.02083333333333333218, 0.03125000000000000000, 0.04166666666666666435, 0.05208333333333333565, 0.06250000000000000000, 0.07291666666666667129, 0.08333333333333332871, 0.09375000000000000000, 0.1041666666666666713, 0.1145833333333333287, 0.1250000000000000000, 0.1354166666666666574, 0.1458333333333333426, 0.1562500000000000000, 0.1666666666666666574, 0.1770833333333333426, 0.1875000000000000000, 0.1979166666666666574, 0.2083333333333333426, 0.2187500000000000000, 0.2291666666666666574, 0.2395833333333333426, 0.2500000000000000000, 0.2604166666666666852, 0.2708333333333333148, 0.2812500000000000000, 0.2916666666666666852, 0.3020833333333333148, 0.3125000000000000000, 0.3229166666666666852, 0.3333333333333333148, 0.3437500000000000000, 0.3541666666666666852, 0.3645833333333333148, 0.3750000000000000000, 0.3854166666666666852, 0.3958333333333333148, 0.4062500000000000000, 0.4166666666666666852, 0.4270833333333333148, 0.4375000000000000000, 0.4479166666666666852, 0.4583333333333333148, 0.4687500000000000000, 0.4791666666666666852, 0.4895833333333333148, 0.5000000000000000000, 0.5104166666666666297, 0.5208333333333333703, 0.5312500000000000000, 0.5416666666666666297, 0.5520833333333333703, 0.5625000000000000000, 0.5729166666666666297, 0.5833333333333333703, 0.5937500000000000000, 0.6041666666666666297, 0.6145833333333333703, 0.6250000000000000000, 0.6354166666666666297, 0.6458333333333333703, 0.6562500000000000000, 0.6666666666666666297, 0.6770833333333333703, 0.6875000000000000000, 0.6979166666666666297, 0.7083333333333333703, 0.7187500000000000000, 0.7291666666666666297, 0.7395833333333333703, 0.7500000000000000000, 0.7604166666666666297, 0.7708333333333333703, 0.7812500000000000000, 0.7916666666666666297, 0.8020833333333333703, 0.8125000000000000000, 0.8229166666666666297, 0.8333333333333333703, 0.8437500000000000000, 0.8541666666666666297, 0.8645833333333333703, 0.8750000000000000000, 0.8854166666666666297, 0.8958333333333333703, 0.9062500000000000000, 0.9166666666666666297, 0.9270833333333333703, 0.9375000000000000000, 0.9448587001587775980 ),
 .UNSPECIFIED. ) 
 GEOMETRIC_REPRESENTATION_ITEM ( )  RATIONAL_B_SPLINE_SURFACE ( (
 ( 1.000000000000000000, 0.9238795325112867385, 1.000000000000000000, 0.9238795325112867385, 1.000000000000000000, 0.9238795325112867385, 1.000000000000000000, 0.9238795325112867385, 1.000000000000000000, 0.9238795325112867385, 1.000000000000000000, 0.9238795325112867385, 1.000000000000000000, 0.9238795325112867385, 1.000000000000000000, 0.9238795325112867385, 1.000000000000000000, 0.9238795325112867385, 1.000000000000000000, 0.9238795325112867385, 1.000000000000000000, 0.9238795325112867385, 1.000000000000000000, 0.9238795325112867385, 1.000000000000000000, 0.9238795325112867385, 1.000000000000000000, 0.9238795325112867385, 1.000000000000000000, 0.9238795325112867385, 1.000000000000000000, 0.9238795325112867385, 1.000000000000000000, 0.9238795325112867385, 1.000000000000000000, 0.9238795325112867385, 1.000000000000000000, 0.9238795325112867385, 1.000000000000000000, 0.9238795325112867385, 1.000000000000000000, 0.9238795325112867385, 1.000000000000000000, 0.9238795325112867385, 1.000000000000000000, 0.9238795325112867385, 1.000000000000000000, 0.9238795325112867385, 1.000000000000000000, 0.9238795325112867385, 1.000000000000000000, 0.9238795325112867385, 1.000000000000000000, 0.9238795325112867385, 1.000000000000000000, 0.9238795325112867385, 1.000000000000000000, 0.9238795325112867385, 1.000000000000000000, 0.9238795325112867385, 1.000000000000000000, 0.9238795325112867385, 1.000000000000000000, 0.9238795325112867385, 1.000000000000000000, 0.9238795325112867385, 1.000000000000000000, 0.9238795325112867385, 1.000000000000000000, 0.9238795325112867385, 1.000000000000000000, 0.9238795325112867385, 1.000000000000000000, 0.9238795325112867385, 1.000000000000000000, 0.9238795325112867385, 1.000000000000000000, 0.9238795325112867385, 1.000000000000000000, 0.9238795325112867385, 1.000000000000000000, 0.9238795325112867385, 1.000000000000000000, 0.9238795325112867385, 1.000000000000000000, 0.9238795325112867385, 1.000000000000000000, 0.9238795325112867385, 1.000000000000000000, 0.9238795325112867385, 1.000000000000000000, 0.9238795325112867385, 1.000000000000000000, 0.9238795325112867385, 1.000000000000000000, 0.9238795325112867385, 1.000000000000000000, 0.9238795325112867385, 1.000000000000000000, 0.9238795325112867385, 1.000000000000000000, 0.9238795325112867385, 1.000000000000000000, 0.9238795325112867385, 1.000000000000000000, 0.9238795325112867385, 1.000000000000000000, 0.9238795325112867385, 1.000000000000000000, 0.9238795325112867385, 1.000000000000000000, 0.9238795325112867385, 1.000000000000000000, 0.9238795325112867385, 1.000000000000000000, 0.9238795325112867385, 1.000000000000000000, 0.9238795325112867385, 1.000000000000000000, 0.9238795325112867385, 1.000000000000000000, 0.9238795325112867385, 1.000000000000000000, 0.9238795325112867385, 1.000000000000000000, 0.9238795325112867385, 1.000000000000000000, 0.9238795325112867385, 1.000000000000000000, 0.9238795325112867385, 1.000000000000000000, 0.9238795325112867385, 1.000000000000000000, 0.9238795325112867385, 1.000000000000000000, 0.9238795325112867385, 1.000000000000000000, 0.9238795325112867385, 1.000000000000000000, 0.9238795325112867385, 1.000000000000000000, 0.9238795325112867385, 1.000000000000000000, 0.9238795325112867385, 1.000000000000000000, 0.9238795325112867385, 1.000000000000000000, 0.9238795325112867385, 1.000000000000000000, 0.9238795325112867385, 1.000000000000000000, 0.9238795325112867385, 1.000000000000000000, 0.9238795325112867385, 1.000000000000000000, 0.9238795325112867385, 1.000000000000000000, 0.9238795325112867385, 1.000000000000000000, 0.9238795325112867385, 1.000000000000000000, 0.9238795325112867385, 1.000000000000000000, 0.9238795325112867385, 1.000000000000000000, 0.9238795325112867385, 1.000000000000000000, 0.9238795325112867385, 1.000000000000000000, 0.9238795325112867385, 1.000000000000000000, 0.9238795325112867385, 1.000000000000000000, 0.9238795325112867385, 1.000000000000000000, 0.9238795325112867385, 1.000000000000000000, 0.9238795325112867385, 1.000000000000000000, 0.9238795325112867385, 1.000000000000000000, 0.9462258211652395667, 0.9684275895297407288),
 ( 1.000000000000000000, 0.9238795325112867385, 1.000000000000000000, 0.9238795325112867385, 1.000000000000000000, 0.9238795325112867385, 1.000000000000000000, 0.9238795325112867385, 1.000000000000000000, 0.9238795325112867385, 1.000000000000000000, 0.9238795325112867385, 1.000000000000000000, 0.9238795325112867385, 1.000000000000000000, 0.9238795325112867385, 1.000000000000000000, 0.9238795325112867385, 1.000000000000000000, 0.9238795325112867385, 1.000000000000000000, 0.9238795325112867385, 1.000000000000000000, 0.9238795325112867385, 1.000000000000000000, 0.9238795325112867385, 1.000000000000000000, 0.9238795325112867385, 1.000000000000000000, 0.9238795325112867385, 1.000000000000000000, 0.9238795325112867385, 1.000000000000000000, 0.9238795325112867385, 1.000000000000000000, 0.9238795325112867385, 1.000000000000000000, 0.9238795325112867385, 1.000000000000000000, 0.9238795325112867385, 1.000000000000000000, 0.9238795325112867385, 1.000000000000000000, 0.9238795325112867385, 1.000000000000000000, 0.9238795325112867385, 1.000000000000000000, 0.9238795325112867385, 1.000000000000000000, 0.9238795325112867385, 1.000000000000000000, 0.9238795325112867385, 1.000000000000000000, 0.9238795325112867385, 1.000000000000000000, 0.9238795325112867385, 1.000000000000000000, 0.9238795325112867385, 1.000000000000000000, 0.9238795325112867385, 1.000000000000000000, 0.9238795325112867385, 1.000000000000000000, 0.9238795325112867385, 1.000000000000000000, 0.9238795325112867385, 1.000000000000000000, 0.9238795325112867385, 1.000000000000000000, 0.9238795325112867385, 1.000000000000000000, 0.9238795325112867385, 1.000000000000000000, 0.9238795325112867385, 1.000000000000000000, 0.9238795325112867385, 1.000000000000000000, 0.9238795325112867385, 1.000000000000000000, 0.9238795325112867385, 1.000000000000000000, 0.9238795325112867385, 1.000000000000000000, 0.9238795325112867385, 1.000000000000000000, 0.9238795325112867385, 1.000000000000000000, 0.9238795325112867385, 1.000000000000000000, 0.9238795325112867385, 1.000000000000000000, 0.9238795325112867385, 1.000000000000000000, 0.9238795325112867385, 1.000000000000000000, 0.9238795325112867385, 1.000000000000000000, 0.9238795325112867385, 1.000000000000000000, 0.9238795325112867385, 1.000000000000000000, 0.9238795325112867385, 1.000000000000000000, 0.9238795325112867385, 1.000000000000000000, 0.9238795325112867385, 1.000000000000000000, 0.9238795325112867385, 1.000000000000000000, 0.9238795325112867385, 1.000000000000000000, 0.9238795325112867385, 1.000000000000000000, 0.9238795325112867385, 1.000000000000000000, 0.9238795325112867385, 1.000000000000000000, 0.9238795325112867385, 1.000000000000000000, 0.9238795325112867385, 1.000000000000000000, 0.9238795325112867385, 1.000000000000000000, 0.9238795325112867385, 1.000000000000000000, 0.9238795325112867385, 1.000000000000000000, 0.9238795325112867385, 1.000000000000000000, 0.9238795325112867385, 1.000000000000000000, 0.9238795325112867385, 1.000000000000000000, 0.9238795325112867385, 1.000000000000000000, 0.9238795325112867385, 1.000000000000000000, 0.9238795325112867385, 1.000000000000000000, 0.9238795325112867385, 1.000000000000000000, 0.9238795325112867385, 1.000000000000000000, 0.9238795325112867385, 1.000000000000000000, 0.9238795325112867385, 1.000000000000000000, 0.9238795325112867385, 1.000000000000000000, 0.9238795325112867385, 1.000000000000000000, 0.9238795325112867385, 1.000000000000000000, 0.9238795325112867385, 1.000000000000000000, 0.9238795325112867385, 1.000000000000000000, 0.9238795325112867385, 1.000000000000000000, 0.9238795325112867385, 1.000000000000000000, 0.9238795325112867385, 1.000000000000000000, 0.9238795325112867385, 1.000000000000000000, 0.9238795325112867385, 1.000000000000000000, 0.9238795325112867385, 1.000000000000000000, 0.9238795325112867385, 1.000000000000000000, 0.9238795325112867385, 1.000000000000000000, 0.9238795325112867385, 1.000000000000000000, 0.9238795325112867385, 1.000000000000000000, 0.9238795325112867385, 1.000000000000000000, 0.9238795325112867385, 1.000000000000000000, 0.9462258211652395667, 0.9684275895297407288) ) ) 
 REPRESENTATION_ITEM ( '' )  SURFACE ( )  );
#21904=VERTEX_POINT ( 'NONE', #25316 ) ;
#21908=CARTESIAN_POINT ( 'NONE',  ( 2.414731522848535132E-15, 39.95820312608393010, 13.14518615778179544 ) ) ;
#21936=CARTESIAN_POINT ( 'NONE',  ( 9.598844408820456309, 36.73359374999999716, -9.598844408820458085 ) ) ;
#21938=CARTESIAN_POINT ( 'NONE',  ( -8.049105076161786076E-16, 37.37851562608393863, -13.14518615778179544 ) ) ;
#21957=CARTESIAN_POINT ( 'NONE',  ( 5.622872871577924592, 32.61601562716786873, 13.57481594606299957 ) ) ;
#21960=CARTESIAN_POINT ( 'NONE',  ( -13.14518615778179722, 32.76484375108393010, -5.444914386472297529 ) ) ;
#21961=CARTESIAN_POINT ( 'NONE',  ( 13.14518615778179900, 40.30546875108393579, 5.444914386472293977 ) ) ;
#21971=CARTESIAN_POINT ( 'NONE',  ( -13.57481594606304398, 34.69960937499999432, 5.622872871577880183 ) ) ;
#21985=ORIENTED_EDGE ( 'NONE', *, *, #3565, .F. ) ;
#21990=VERTEX_POINT ( 'NONE', #24905 ) ;
#21992=CARTESIAN_POINT ( 'NONE',  ( -5.444914386472299306, 39.11484375108394573, 13.14518615778179722 ) ) ;
#22027=DIRECTION ( 'NONE',  ( 0.000000000000000000, 1.000000000000000000, 0.000000000000000000 ) ) ;
#22041=CARTESIAN_POINT ( 'NONE',  ( 5.444914386472302859, 37.62656250108393863, 13.14518615778179189 ) ) ;
#22061=EDGE_CURVE ( 'NONE', #18468, #25494, #6484, .T. ) ;
#22063=CARTESIAN_POINT ( 'NONE',  ( 8.193155644910682156, 35.99999999999998579, 10.45682415286346512 ) ) ;
#22067=CIRCLE ( 'NONE', #24317, 1.000000000000000888 ) ;
#22075=CARTESIAN_POINT ( 'NONE',  ( 5.622872871577878406, 36.48554687499999716, 13.57481594606304576 ) ) ;
#22077=CARTESIAN_POINT ( 'NONE',  ( 2.414731522848535132E-15, 38.56914062608393579, 13.14518615778179544 ) ) ;
#22099=CARTESIAN_POINT ( 'NONE',  ( 13.57481594606304576, 32.76484375216787015, -1.662435489736055892E-15 ) ) ;
#22104=CARTESIAN_POINT ( 'NONE',  ( -13.14518615778179544, 40.75195312608393294, 0.000000000000000000 ) ) ;
#22143=VERTEX_POINT ( 'NONE', #12458 ) ;
#22153=B_SPLINE_CURVE_WITH_KNOTS ( 'NONE', 3,
 ( #21794, #22214, #2693, #15349, #24065, #4541, #11354, #17642, #26349, #6808, #555, #27067, #9519, #25192, #7370, #7807, #3257, #20646, #18644, #25057, #16497, #1407, #3539, #12195, #18359, #5398, #22787, #18217, #22498, #14346, #12059 ),
 .UNSPECIFIED., .F., .F.,
 ( 4, 2, 2, 2, 2, 2, 2, 2, 2, 2, 1, 2, 2, 2, 2, 4 ),
 ( 0.000000000000000000, 0.001656255954913781435, 0.003312511909827562870, 0.004968767864741344305, 0.005796895842198234589, 0.006625023819655125740, 0.008281279774568908042, 0.009937535729482686875, 0.01325004763931025148, 0.01490630359422403031, 0.01656255954913780915, 0.01821881550405159145, 0.01987507145896537028, 0.02318758336879293835, 0.02484383932370672066, 0.02650009527862050296 ),
 .UNSPECIFIED. ) ;
#22169=CIRCLE ( 'NONE', #14419, 23.26794919243112858 ) ;
#22171=DIRECTION ( 'NONE',  ( -0.000000000000000000, -1.000000000000000000, -0.000000000000000000 ) ) ;
#22181=CARTESIAN_POINT ( 'NONE',  ( -9.295050272127046043, 36.48554687608393721, -9.295050272127046043 ) ) ;
#22194=ADVANCED_FACE ( 'NONE', ( #11026 ), #13480, .F. ) ;
#22201=CARTESIAN_POINT ( 'NONE',  ( 9.432006169634068016, 36.00000000000000711, 9.391769196590193047 ) ) ;
#22205=CARTESIAN_POINT ( 'NONE',  ( -5.622872871577873077, 37.77539062716788010, -13.57481594606304753 ) ) ;
#22213=CARTESIAN_POINT ( 'NONE',  ( 2.493653234604083739E-15, 36.43593749999999432, 13.57481594606304576 ) ) ;
#22214=CARTESIAN_POINT ( 'NONE',  ( 3.628614293284873948, 36.00000000000000711, -13.08307257738123219 ) ) ;
#22216=CARTESIAN_POINT ( 'NONE',  ( 13.14518615778179900, 33.16171875108393863, 5.444914386472293977 ) ) ;
#22219=CARTESIAN_POINT ( 'NONE',  ( -8.312177448680279460E-16, 36.13828125216787157, -13.57481594606304576 ) ) ;
#22230=ORIENTED_EDGE ( 'NONE', *, *, #8596, .F. ) ;
#22241=CARTESIAN_POINT ( 'NONE',  ( 0.000000000000000000, 29.95886589889650509, 0.000000000000000000 ) ) ;
#22245=CARTESIAN_POINT ( 'NONE',  ( 2.414731522848535132E-15, 36.98164062608393721, 13.14518615778179544 ) ) ;
#22270=CARTESIAN_POINT ( 'NONE',  ( 0.000000000000000000, 23.00000000000000000, 25.00000000000001066 ) ) ;
#22279=CARTESIAN_POINT ( 'NONE',  ( 13.14518615778179544, 35.39414062608393152, -1.609821015232357215E-15 ) ) ;
#22282=LINE ( 'NONE', #2472, #14343 ) ;
#22298=CONICAL_SURFACE ( 'NONE', #8632, 25.00000000000000711, 0.5235987755983000369 ) ;
#22326=CARTESIAN_POINT ( 'NONE',  ( 13.14518615778179544, 36.98164062608393010, -1.609821015232357215E-15 ) ) ;
#22337=VERTEX_POINT ( 'NONE', #4640 ) ;
#22338=CARTESIAN_POINT ( 'NONE',  ( -8.312177448680279460E-16, 33.65781249999999147, -13.57481594606304576 ) ) ;
#22346=DIRECTION ( 'NONE',  ( 0.000000000000000000, 1.000000000000000000, 0.000000000000000000 ) ) ;
#22348=CARTESIAN_POINT ( 'NONE',  ( -13.57481594606304576, 39.51171875216787299, 0.000000000000000000 ) ) ;
#22353=CARTESIAN_POINT ( 'NONE',  ( 5.622872871577878406, 35.69179687499999432, 13.57481594606304576 ) ) ;
#22355=CARTESIAN_POINT ( 'NONE',  ( -13.14518615778179900, 34.35234375108393579, -5.444914386472297529 ) ) ;
#22357=CARTESIAN_POINT ( 'NONE',  ( 2.414731522848535132E-15, 35.98945312608393010, 13.14518615778179544 ) ) ;
#22358=AXIS2_PLACEMENT_3D ( 'NONE', #7082, #15780, #24485 ) ;
#22359=CARTESIAN_POINT ( 'NONE',  ( 5.622872871577871301, 35.29492187716788720, -13.57481594606304753 ) ) ;
#22371=CARTESIAN_POINT ( 'NONE',  ( 9.598844408820459861, 34.94765624999999432, 9.598844408820456309 ) ) ;
#22381=ORIENTED_EDGE ( 'NONE', *, *, #11040, .F. ) ;
#22382=CARTESIAN_POINT ( 'NONE',  ( 2.414731522848535132E-15, 36.18789062608393436, 13.14518615778179544 ) ) ;
#22385=EDGE_CURVE ( 'NONE', #15812, #15410, #8041, .T. ) ;
#22416=CARTESIAN_POINT ( 'NONE',  ( -13.14518615778179900, 36.53515625108392584, -5.444914386472297529 ) ) ;
#22440=CARTESIAN_POINT ( 'NONE',  ( 5.622872871577780707, 34.40195312499999858, -13.57481594606313990 ) ) ;
#22456=EDGE_CURVE ( 'NONE', #15410, #15812, #13016, .T. ) ;
#22459=CARTESIAN_POINT ( 'NONE',  ( -8.312177448680279460E-16, 33.75703125216787726, -13.57481594606304576 ) ) ;
#22467=CARTESIAN_POINT ( 'NONE',  ( -5.444914386472299306, 34.35234375108392868, 13.14518615778179722 ) ) ;
#22475=DIRECTION ( 'NONE',  ( -0.5282856486898074300, 0.000000000000000000, 0.8490667072665075699 ) ) ;
#22489=CARTESIAN_POINT ( 'NONE',  ( 2.493653234604083739E-15, 39.71015625216787015, 13.57481594606304576 ) ) ;
#22495=DIRECTION ( 'NONE',  ( -0.000000000000000000, -1.000000000000000000, -0.000000000000000000 ) ) ;
#22497=CARTESIAN_POINT ( 'NONE',  ( 5.622872871577871301, 32.81445312499999289, -13.57481594606304753 ) ) ;
#22498=CARTESIAN_POINT ( 'NONE',  ( -13.17415721692276165, 36.00000000000000000, 0.03826467346021143745 ) ) ;
#22499=CARTESIAN_POINT ( 'NONE',  ( 13.14518615778179544, 34.00507812608393721, -1.609821015232357215E-15 ) ) ;
#22502=CARTESIAN_POINT ( 'NONE',  ( -9.598844408820458085, 34.65000000216787868, -9.598844408820458085 ) ) ;
#22508=VERTEX_POINT ( 'NONE', #8108 ) ;
#22513=ORIENTED_EDGE ( 'NONE', *, *, #16095, .F. ) ;
#22528=CARTESIAN_POINT ( 'NONE',  ( 2.414731522848535132E-15, 35.39414062608393863, 13.14518615778179544 ) ) ;
#22536=CARTESIAN_POINT ( 'NONE',  ( -9.598844408820454532, 34.74921874999999716, 9.598844408820459861 ) ) ;
#22541=AXIS2_PLACEMENT_3D ( 'NONE', #4246, #6381, #113 ) ;
#22562=CARTESIAN_POINT ( 'NONE',  ( 13.14518615778179544, 36.98164062608393010, -1.609821015232357215E-15 ) ) ;
#22581=ORIENTED_EDGE ( 'NONE', *, *, #8760, .F. ) ;
#22583=CARTESIAN_POINT ( 'NONE',  ( 13.57481594606304753, 34.30273437500000000, -5.622872871577873966 ) ) ;
#22615=DIRECTION ( 'NONE',  ( -0.000000000000000000, -1.000000000000000000, -0.000000000000000000 ) ) ;
#22634=CARTESIAN_POINT ( 'NONE',  ( -5.444914386472299306, 32.16953125108393152, 13.14518615778179722 ) ) ;
#22637=DIRECTION ( 'NONE',  ( 0.000000000000000000, 0.000000000000000000, -1.000000000000000000 ) ) ;
#22645=CARTESIAN_POINT ( 'NONE',  ( 13.57481594606304576, 33.45937499999999432, -1.662435489736055892E-15 ) ) ;
#22647=CARTESIAN_POINT ( 'NONE',  ( 13.14518615778179900, 33.26093750108393721, -5.444914386472297529 ) ) ;
#22649=CARTESIAN_POINT ( 'NONE',  ( 13.14518615778179544, 34.60039062608392868, -1.609821015232357215E-15 ) ) ;
#22650=CARTESIAN_POINT ( 'NONE',  ( 9.598844408820456309, 36.83281250216787583, -9.598844408820458085 ) ) ;
#22651=DIRECTION ( 'NONE',  ( -0.000000000000000000, -1.000000000000000000, -0.000000000000000000 ) ) ;
#22655=CARTESIAN_POINT ( 'NONE',  ( -8.312177448680279460E-16, 32.07031249999999289, -13.57481594606304576 ) ) ;
#22662=LINE ( 'NONE', #5416, #12996 ) ;
#22674=CARTESIAN_POINT ( 'NONE',  ( 5.444914386472297529, 34.94765625108394147, -13.14518615778179900 ) ) ;
#22705=CARTESIAN_POINT ( 'NONE',  ( -8.049105076161786076E-16, 37.97382812608393721, -13.14518615778179544 ) ) ;
#22715=EDGE_CURVE ( 'NONE', #18166, #15854, #2901, .T. ) ;
#22726=CARTESIAN_POINT ( 'NONE',  ( 9.598844408820456309, 34.35234374999999574, -9.598844408820458085 ) ) ;
#22752=CARTESIAN_POINT ( 'NONE',  ( -13.57481594606304753, 35.49335937716787726, -5.622872871577872189 ) ) ;
#22754=CARTESIAN_POINT ( 'NONE',  ( 0.000000000000000000, 23.00000000000000000, 0.000000000000000000 ) ) ;
#22762=FACE_OUTER_BOUND ( 'NONE', #16638, .T. ) ;
#22778=CARTESIAN_POINT ( 'NONE',  ( -9.598844408820454532, 38.02343750216788010, 9.598844408820459861 ) ) ;
#22786=CARTESIAN_POINT ( 'NONE',  ( -5.622872871577873077, 33.21132812499999432, 13.57481594606304753 ) ) ;
#22787=CARTESIAN_POINT ( 'NONE',  ( -13.10247082172194943, 36.00000000000000711, -1.608626461598226420 ) ) ;
#22788=CARTESIAN_POINT ( 'NONE',  ( 13.14518615778179544, 34.79882812608394005, -1.609821015232357215E-15 ) ) ;
#22792=CARTESIAN_POINT ( 'NONE',  ( -13.57481594606304576, 35.59257812716788294, 5.622872871577880183 ) ) ;
#22797=FACE_OUTER_BOUND ( 'NONE', #7158, .T. ) ;
#22815=CARTESIAN_POINT ( 'NONE',  ( -13.14518615778179900, 36.73359375108393010, -5.444914386472297529 ) ) ;
#22831=VECTOR ( 'NONE', #18706, 1000.000000000000000 ) ;
#22840=CARTESIAN_POINT ( 'NONE',  ( 1.137167824541903460, 36.00000000000000000, 13.09590655363594180 ) ) ;
#22845=ORIENTED_EDGE ( 'NONE', *, *, #16501, .F. ) ;
#22847=CARTESIAN_POINT ( 'NONE',  ( -13.14518615778179544, 36.58476562608393579, 0.000000000000000000 ) ) ;
#22895=CARTESIAN_POINT ( 'NONE',  ( -13.14518615778179900, 39.11484375108394573, -5.444914386472297529 ) ) ;
#22912=CARTESIAN_POINT ( 'NONE',  ( 2.414731522848535132E-15, 32.21914062608393436, 13.14518615778179544 ) ) ;
#22916=( NAMED_UNIT ( * ) SI_UNIT ( $, .STERADIAN. ) SOLID_ANGLE_UNIT ( ) );
#22925=CARTESIAN_POINT ( 'NONE',  ( 13.57481594606304753, 33.50898437499999716, -5.622872871577873077 ) ) ;
#22928=CARTESIAN_POINT ( 'NONE',  ( -5.622872871577873077, 39.56132812499999574, 13.57481594606304753 ) ) ;
#22930=CARTESIAN_POINT ( 'NONE',  ( -8.049105076161786076E-16, 34.79882812608393294, -13.14518615778179544 ) ) ;
#22931=CARTESIAN_POINT ( 'NONE',  ( -8.312177448680279460E-16, 33.75703125216787726, -13.57481594606304576 ) ) ;
#22935=CARTESIAN_POINT ( 'NONE',  ( 1.662435489736055892E-15, 36.00000000000000000, 13.57481594606304576 ) ) ;
#22936=CARTESIAN_POINT ( 'NONE',  ( -8.312177448680279460E-16, 35.34453125216787583, -13.57481594606304576 ) ) ;
#22942=ORIENTED_EDGE ( 'NONE', *, *, #24186, .F. ) ;
#22957=CARTESIAN_POINT ( 'NONE',  ( 2.414731522848535132E-15, 33.80664062608393294, 13.14518615778179544 ) ) ;
#22986=CARTESIAN_POINT ( 'NONE',  ( -13.14518615778179189, 32.66562500108393863, 5.444914386472304635 ) ) ;
#22992=DIRECTION ( 'NONE',  ( -0.000000000000000000, -1.000000000000000000, -0.000000000000000000 ) ) ;
#22996=CARTESIAN_POINT ( 'NONE',  ( -13.14518615778179189, 35.04687500108393294, 5.444914386472304635 ) ) ;
#23027=LINE ( 'NONE', #13740, #14332 ) ;
#23030=CARTESIAN_POINT ( 'NONE',  ( 5.622872871577961895, 34.50117187716787726, -13.57481594606295339 ) ) ;
#23032=CARTESIAN_POINT ( 'NONE',  ( 9.295050272127046043, 39.66054687608393436, -9.295050272127046043 ) ) ;
#23039=ORIENTED_EDGE ( 'NONE', *, *, #14844, .T. ) ;
#23040=CARTESIAN_POINT ( 'NONE',  ( 7.171391216998964424, 31.99955315621561525, -11.52591757658528948 ) ) ;
#23062=CARTESIAN_POINT ( 'NONE',  ( -13.57481594606304753, 39.36289062499999858, -5.622872871577873077 ) ) ;
#23063=CARTESIAN_POINT ( 'NONE',  ( -13.14518615778179722, 32.56640625108394005, -5.444914386472297529 ) ) ;
#23064=CARTESIAN_POINT ( 'NONE',  ( -13.57481594606304753, 32.31835937716786589, -5.622872871577873077 ) ) ;
#23089=CARTESIAN_POINT ( 'NONE',  ( -13.14518615778179544, 32.81445312608393294, 0.000000000000000000 ) ) ;
#23109=CARTESIAN_POINT ( 'NONE',  ( 0.2703369776648356093, 36.00000000000000000, 13.14949859323919590 ) ) ;
#23115=CARTESIAN_POINT ( 'NONE',  ( -9.598844408820458085, 31.47500000216787441, -9.598844408820458085 ) ) ;
#23123=CARTESIAN_POINT ( 'NONE',  ( -13.14518615778179189, 31.87187500108393223, 5.444914386472304635 ) ) ;
#23136=CARTESIAN_POINT ( 'NONE',  ( -13.14518615778179544, 35.79101562608393294, 0.000000000000000000 ) ) ;
#23145=DIRECTION ( 'NONE',  ( 0.000000000000000000, 1.000000000000000000, 0.000000000000000000 ) ) ;
#23168=CARTESIAN_POINT ( 'NONE',  ( 9.598844408820459861, 34.25312500216787015, 9.598844408820456309 ) ) ;
#23170=CARTESIAN_POINT ( 'NONE',  ( -9.295050272127046043, 39.85898437608393152, -9.295050272127046043 ) ) ;
#23174=CARTESIAN_POINT ( 'NONE',  ( -8.312177448680279460E-16, 32.96328125216787441, -13.57481594606304576 ) ) ;
#23195=PLANE ( 'NONE',  #25651 ) ;
#23202=CARTESIAN_POINT ( 'NONE',  ( -8.312177448680279460E-16, 33.75703125216787726, -13.57481594606304576 ) ) ;
#23204=CARTESIAN_POINT ( 'NONE',  ( -13.57481594606304753, 40.95039062499999005, -5.622872871577873077 ) ) ;
#23205=CARTESIAN_POINT ( 'NONE',  ( -8.049105076161786076E-16, 33.21132812608393436, -13.14518615778179544 ) ) ;
#23206=CARTESIAN_POINT ( 'NONE',  ( -8.312177448680279460E-16, 32.96328125216787441, -13.57481594606304576 ) ) ;
#23212=FACE_OUTER_BOUND ( 'NONE', #14704, .T. ) ;
#23228=CARTESIAN_POINT ( 'NONE',  ( -9.295050272127044266, 32.91367187608393152, 9.295050272127047819 ) ) ;
#23230=DIRECTION ( 'NONE',  ( 0.000000000000000000, 0.000000000000000000, 1.000000000000000000 ) ) ;
#23258=ADVANCED_FACE ( 'NONE', ( #27611, #20638 ), #23195, .T. ) ;
#23259=EDGE_LOOP ( 'NONE', ( #18269, #16928, #5871, #3127 ) ) ;
#23261=CARTESIAN_POINT ( 'NONE',  ( -13.14518615778179544, 34.20351562608393436, 0.000000000000000000 ) ) ;
#23268=EDGE_LOOP ( 'NONE', ( #15134, #6787, #5197, #23402, #25244, #26841, #22581, #10539 ) ) ;
#23277=CARTESIAN_POINT ( 'NONE',  ( -13.14518615778179544, 34.20351562608393436, 0.000000000000000000 ) ) ;
#23334=CARTESIAN_POINT ( 'NONE',  ( -13.57481594606304576, 32.26874999999999716, 0.000000000000000000 ) ) ;
#23336=CARTESIAN_POINT ( 'NONE',  ( 0.000000000000000000, 36.00000000000000000, 0.000000000000000000 ) ) ;
#23337=CARTESIAN_POINT ( 'NONE',  ( -9.295050272127044266, 32.11992187608393579, 9.295050272127047819 ) ) ;
#23338=CARTESIAN_POINT ( 'NONE',  ( -9.295050272127044266, 33.50898437608393010, 9.295050272127047819 ) ) ;
#23340=CARTESIAN_POINT ( 'NONE',  ( -13.57481594606304753, 31.52460937716787370, -5.622872871577873077 ) ) ;
#23363=CARTESIAN_POINT ( 'NONE',  ( -9.295050272127046043, 31.92148437608393508, -9.295050272127046043 ) ) ;
#23394=CARTESIAN_POINT ( 'NONE',  ( -5.444914386472297529, 35.04687500108393294, -13.14518615778179722 ) ) ;
#23395=CARTESIAN_POINT ( 'NONE',  ( -13.14518615778179544, 32.61601562608393579, 0.000000000000000000 ) ) ;
#23402=ORIENTED_EDGE ( 'NONE', *, *, #20623, .F. ) ;
#23411=CARTESIAN_POINT ( 'NONE',  ( 13.14518615778179900, 33.85625000108393579, -5.444914386472297529 ) ) ;
#23446=CIRCLE ( 'NONE', #22541, 16.91709623134523000 ) ;
#23447=DIRECTION ( 'NONE',  ( 0.000000000000000000, 1.000000000000000000, 0.000000000000000000 ) ) ;
#23474=DIRECTION ( 'NONE',  ( 0.000000000000000000, 0.000000000000000000, -1.000000000000000000 ) ) ;
#23475=CARTESIAN_POINT ( 'NONE',  ( 5.622872871577871301, 40.75195312500000711, -13.57481594606304753 ) ) ;
#23476=CARTESIAN_POINT ( 'NONE',  ( -13.14518615778179189, 32.66562500108393863, 5.444914386472304635 ) ) ;
#23477=CARTESIAN_POINT ( 'NONE',  ( 13.57481594606304931, 32.71523437716787441, 5.622872871577869525 ) ) ;
#23524=CARTESIAN_POINT ( 'NONE',  ( -5.622872871577965448, 31.72304687716787086, 13.57481594606295161 ) ) ;
#23529=AXIS2_PLACEMENT_3D ( 'NONE', #1348, #23145, #3620 ) ;
#23533=ORIENTED_EDGE ( 'NONE', *, *, #14737, .T. ) ;
#23534=CARTESIAN_POINT ( 'NONE',  ( -8.049105076161786076E-16, 34.20351562608394147, -13.14518615778179544 ) ) ;
#23535=CARTESIAN_POINT ( 'NONE',  ( 9.295050272127047819, 34.50117187608393010, 9.295050272127046043 ) ) ;
#23552=CARTESIAN_POINT ( 'NONE',  ( 13.14518615778179544, 32.21914062608393436, -1.609821015232357215E-15 ) ) ;
#23572=CARTESIAN_POINT ( 'NONE',  ( -9.598844408820454532, 34.84843750216787583, 9.598844408820459861 ) ) ;
#23578=LINE ( 'NONE', #6058, #2141 ) ;
#23582=DIRECTION ( 'NONE',  ( -0.000000000000000000, -1.000000000000000000, -0.000000000000000000 ) ) ;
#23586=ORIENTED_EDGE ( 'NONE', *, *, #27480, .F. ) ;
#23608=DIRECTION ( 'NONE',  ( 1.000000000000000000, 0.000000000000000000, 0.000000000000000000 ) ) ;
#23615=CARTESIAN_POINT ( 'NONE',  ( -5.444914386472299306, 32.76484375108393010, 13.14518615778179722 ) ) ;
#23617=CARTESIAN_POINT ( 'NONE',  ( 9.295050272127046043, 40.25585937608393294, -9.295050272127046043 ) ) ;
#23637=VECTOR ( 'NONE', #27975, 1000.000000000000000 ) ;
#23649=CARTESIAN_POINT ( 'NONE',  ( 9.295050272127046043, 38.86679687608393863, -9.295050272127046043 ) ) ;
#23659=CARTESIAN_POINT ( 'NONE',  ( -6.338290792349636327, 36.00000000000000000, 11.53992004315014164 ) ) ;
#23662=ORIENTED_EDGE ( 'NONE', *, *, #19418, .F. ) ;
#23673=CARTESIAN_POINT ( 'NONE',  ( -13.14518615778179544, 35.98945312608393721, 0.000000000000000000 ) ) ;
#23674=( BOUNDED_CURVE ( )  B_SPLINE_CURVE ( 2, ( #4053, #8455, #23572, #13129, #10996, #8597, #6457, #4187, #8312 ),
 .UNSPECIFIED., .F., .F. ) 
 B_SPLINE_CURVE_WITH_KNOTS ( ( 3, 2, 2, 2, 3 ),
 ( 0.5624999999999996669, 0.5729166666666664076, 0.5833333333333332593, 0.5937500000000001110, 0.6041666666666668517 ),
 .UNSPECIFIED. ) 
 CURVE ( )  GEOMETRIC_REPRESENTATION_ITEM ( )  RATIONAL_B_SPLINE_CURVE ( ( 1.000000000000002442, 0.9238795325112842960, 1.000000000000000000, 0.9238795325112867385, 1.000000000000000000, 0.9238795325112867385, 1.000000000000000000, 0.9238795325112850731, 1.000000000000001554 ) ) 
 REPRESENTATION_ITEM ( '' )  );
#23675=CARTESIAN_POINT ( 'NONE',  ( 13.14518615778179544, 37.97382812608393721, -1.609821015232357215E-15 ) ) ;
#23692=CARTESIAN_POINT ( 'NONE',  ( -5.444914386472297529, 32.46718750108393436, -13.14518615778179900 ) ) ;
#23702=CARTESIAN_POINT ( 'NONE',  ( 0.000000000000000000, 36.00000000000000000, 0.000000000000000000 ) ) ;
#23707=CARTESIAN_POINT ( 'NONE',  ( -13.14518615778179544, 38.96601562608393721, 0.000000000000000000 ) ) ;
#23728=DIRECTION ( 'NONE',  ( 0.000000000000000000, 0.000000000000000000, -1.000000000000000000 ) ) ;
#23730=EDGE_LOOP ( 'NONE', ( #13249, #10958, #22513, #963 ) ) ;
#23752=CARTESIAN_POINT ( 'NONE',  ( -9.295050272127044266, 38.27148437608393294, 9.295050272127047819 ) ) ;
#23765=EDGE_CURVE ( 'NONE', #15725, #15812, #2649, .T. ) ;
#23770=CARTESIAN_POINT ( 'NONE',  ( 1.137167824541903460, 36.00000000000000000, 13.09590655363594180 ) ) ;
#23780=CARTESIAN_POINT ( 'NONE',  ( 13.57481594606304576, 36.63437499999999858, -1.662435489736055892E-15 ) ) ;
#23783=CARTESIAN_POINT ( 'NONE',  ( 9.295050272127047819, 36.28710937608393294, 9.295050272127046043 ) ) ;
#23788=DIRECTION ( 'NONE',  ( 0.000000000000000000, 0.000000000000000000, -1.000000000000000000 ) ) ;
#23808=CARTESIAN_POINT ( 'NONE',  ( 13.14518615778179722, 34.84843750108393579, -5.444914386472297529 ) ) ;
#23809=CARTESIAN_POINT ( 'NONE',  ( -13.14518615778179900, 40.70234375108393721, -5.444914386472297529 ) ) ;
#23828=CARTESIAN_POINT ( 'NONE',  ( -5.444914386472297529, 31.67343750108393863, -13.14518615778179900 ) ) ;
#23839=DIRECTION ( 'NONE',  ( 0.000000000000000000, 0.000000000000000000, -1.000000000000000000 ) ) ;
#23848=CARTESIAN_POINT ( 'NONE',  ( -13.57481594606304576, 33.85624999999999574, 0.000000000000000000 ) ) ;
#23866=AXIS2_PLACEMENT_3D ( 'NONE', #18121, #7282, #18271 ) ;
#23885=CONICAL_SURFACE ( 'NONE', #26630, 19.22649730810373470, 0.5235987755983000369 ) ;
#23892=CARTESIAN_POINT ( 'NONE',  ( -13.14518615778179544, 38.17226562608393436, 0.000000000000000000 ) ) ;
#23909=CARTESIAN_POINT ( 'NONE',  ( 12.66784425494596000, 35.99999999999998579, 4.396229039743023037 ) ) ;
#23923=CARTESIAN_POINT ( 'NONE',  ( -9.598844408820454532, 37.13046874999999147, 9.598844408820459861 ) ) ;
#23925=CARTESIAN_POINT ( 'NONE',  ( 13.14518615778179544, 37.97382812608393721, -1.609821015232357215E-15 ) ) ;
#23937=ORIENTED_EDGE ( 'NONE', *, *, #17851, .T. ) ;
#23950=CARTESIAN_POINT ( 'NONE',  ( 5.444914386472297529, 34.94765625108394147, -13.14518615778179722 ) ) ;
#23951=CARTESIAN_POINT ( 'NONE',  ( 9.295050272127047819, 38.66835937608393436, 9.295050272127046043 ) ) ;
#23965=DIRECTION ( 'NONE',  ( 0.000000000000000000, 1.000000000000000000, 0.000000000000000000 ) ) ;
#23986=CARTESIAN_POINT ( 'NONE',  ( -8.049105076161786076E-16, 39.56132812608393579, -13.14518615778179544 ) ) ;
#23997=ORIENTED_EDGE ( 'NONE', *, *, #88, .F. ) ;
#24028=DIRECTION ( 'NONE',  ( 0.000000000000000000, 0.000000000000000000, 1.000000000000000000 ) ) ;
#24033=CARTESIAN_POINT ( 'NONE',  ( -9.295050272127046043, 39.66054687608393436, -9.295050272127046043 ) ) ;
#24041=CARTESIAN_POINT ( 'NONE',  ( -2.407595600654690178E-15, 10.00000000000000178, -16.91709623134523000 ) ) ;
#24063=CARTESIAN_POINT ( 'NONE',  ( -5.622872871577873077, 36.38632812499999858, 13.57481594606304753 ) ) ;
#24065=CARTESIAN_POINT ( 'NONE',  ( 1.464337720320554093, 36.00000000000002842, -13.46163418879032037 ) ) ;
#24066=CARTESIAN_POINT ( 'NONE',  ( -13.14518615778179900, 37.52734375108393294, -5.444914386472297529 ) ) ;
#24093=CARTESIAN_POINT ( 'NONE',  ( 9.295050272127046043, 38.07304687608393579, -9.295050272127046043 ) ) ;
#24122=DIRECTION ( 'NONE',  ( -0.000000000000000000, -1.000000000000000000, -0.000000000000000000 ) ) ;
#24128=CARTESIAN_POINT ( 'NONE',  ( 9.295050272127046043, 38.66835937608393436, -9.295050272127046043 ) ) ;
#24147=DIRECTION ( 'NONE',  ( -0.000000000000000000, -1.000000000000000000, -0.000000000000000000 ) ) ;
#24157=ADVANCED_FACE ( 'NONE', ( #17071 ), #16672, .T. ) ;
#24177=CARTESIAN_POINT ( 'NONE',  ( 9.295050272127046043, 37.87460937608393152, -9.295050272127046043 ) ) ;
#24182=DIRECTION ( 'NONE',  ( -0.000000000000000000, -1.000000000000000000, -0.000000000000000000 ) ) ;
#24186=EDGE_CURVE ( 'NONE', #12537, #21429, #6048, .T. ) ;
#24205=CARTESIAN_POINT ( 'NONE',  ( -9.598844408820458085, 32.26875000216787726, -9.598844408820458085 ) ) ;
#24206=CARTESIAN_POINT ( 'NONE',  ( -9.598844408820458085, 36.93203124999999432, -9.598844408820458085 ) ) ;
#24209=CARTESIAN_POINT ( 'NONE',  ( -5.444914386472299306, 37.72578125108395142, 13.14518615778179722 ) ) ;
#24213=FACE_OUTER_BOUND ( 'NONE', #23268, .T. ) ;
#24232=CARTESIAN_POINT ( 'NONE',  ( 5.444914386472297529, 32.56640625108394005, -13.14518615778179722 ) ) ;
#24233=CARTESIAN_POINT ( 'NONE',  ( 5.444914386472297529, 38.91640625108393436, -13.14518615778179900 ) ) ;
#24242=CARTESIAN_POINT ( 'NONE',  ( -5.622872871577964560, 34.50117187499998295, -13.57481594606295339 ) ) ;
#24265=CARTESIAN_POINT ( 'NONE',  ( 13.14518615778179900, 39.31328125108392868, 5.444914386472293977 ) ) ;
#24284=CARTESIAN_POINT ( 'NONE',  ( 5.622872871577786924, 34.10429687500000284, 13.57481594606313813 ) ) ;
#24296=ORIENTED_EDGE ( 'NONE', *, *, #5776, .T. ) ;
#24310=EDGE_CURVE ( 'NONE', #27857, #11809, #7300, .T. ) ;
#24311=CARTESIAN_POINT ( 'NONE',  ( 13.14518615778179900, 36.23750000108393010, -5.444914386472297529 ) ) ;
#24317=AXIS2_PLACEMENT_3D ( 'NONE', #20264, #750, #11689 ) ;
#24325=CARTESIAN_POINT ( 'NONE',  ( 13.57481594606304931, 33.40976562499999858, 5.622872871577868636 ) ) ;
#24337=CARTESIAN_POINT ( 'NONE',  ( 5.622872871577878406, 38.17226562716786731, 13.57481594606304576 ) ) ;
#24342=CARTESIAN_POINT ( 'NONE',  ( 9.598844408820459861, 37.32890624999999574, 9.598844408820456309 ) ) ;
#24344=CARTESIAN_POINT ( 'NONE',  ( -5.444914386472299306, 33.75703125108393721, 13.14518615778179722 ) ) ;
#24360=CARTESIAN_POINT ( 'NONE',  ( 5.622872871577961895, 35.19570312499999432, -13.57481594606295339 ) ) ;
#24371=CARTESIAN_POINT ( 'NONE',  ( -9.295050272127044266, 35.29492187608393294, 9.295050272127047819 ) ) ;
#24375=CARTESIAN_POINT ( 'NONE',  ( -5.622872871577965448, 32.41757812499999858, 13.57481594606295161 ) ) ;
#24379=VECTOR ( 'NONE', #6191, 1000.000000000000114 ) ;
#24395=CYLINDRICAL_SURFACE ( 'NONE', #25732, 13.57481594606304576 ) ;
#24404=CARTESIAN_POINT ( 'NONE',  ( -13.14518615778179544, 35.79101562608393294, 0.000000000000000000 ) ) ;
#24418=CONICAL_SURFACE ( 'NONE', #8035, 25.00000000000000711, 0.5235987755983000369 ) ;
#24425=CARTESIAN_POINT ( 'NONE',  ( 9.598844408820459861, 34.15390624999999858, 9.598844408820456309 ) ) ;
#24454=CARTESIAN_POINT ( 'NONE',  ( -9.295050272127046043, 34.89804687608393152, -9.295050272127046043 ) ) ;
#24456=DIRECTION ( 'NONE',  ( -0.000000000000000000, -1.000000000000000000, -0.000000000000000000 ) ) ;
#24480=CARTESIAN_POINT ( 'NONE',  ( -9.598844408820454532, 38.81718750216787583, 9.598844408820459861 ) ) ;
#24485=DIRECTION ( 'NONE',  ( 0.000000000000000000, 0.000000000000000000, 1.000000000000000000 ) ) ;
#24488=CARTESIAN_POINT ( 'NONE',  ( 2.493653234604083739E-15, 34.84843749999999574, 13.57481594606304576 ) ) ;
#24490=CARTESIAN_POINT ( 'NONE',  ( 13.14518615778179900, 34.74921875108395142, 5.444914386472293977 ) ) ;
#24493=CARTESIAN_POINT ( 'NONE',  ( 9.598844408820459861, 35.84062500216786873, 9.598844408820456309 ) ) ;
#24518=CARTESIAN_POINT ( 'NONE',  ( 9.295050272127047819, 36.28710937608393294, 9.295050272127046043 ) ) ;
#24527=CARTESIAN_POINT ( 'NONE',  ( -13.57481594606304576, 34.64999999999999147, 0.000000000000000000 ) ) ;
#24548=ORIENTED_EDGE ( 'NONE', *, *, #11040, .T. ) ;
#24550=CARTESIAN_POINT ( 'NONE',  ( 5.444914386472302859, 36.83281250108392868, 13.14518615778179189 ) ) ;
#24590=CARTESIAN_POINT ( 'NONE',  ( -5.622872871577873966, 34.10429687716786873, 13.57481594606304753 ) ) ;
#24603=CARTESIAN_POINT ( 'NONE',  ( -9.295050272127044266, 37.47773437608393010, 9.295050272127047819 ) ) ;
#24614=CARTESIAN_POINT ( 'NONE',  ( 2.493653234604083739E-15, 33.36015625216786873, 13.57481594606304576 ) ) ;
#24626=CARTESIAN_POINT ( 'NONE',  ( 5.622872871577878406, 39.75976562716787299, 13.57481594606304576 ) ) ;
#24634=CARTESIAN_POINT ( 'NONE',  ( 13.57481594606304931, 33.40976562499999858, 5.622872871577869525 ) ) ;
#24636=CARTESIAN_POINT ( 'NONE',  ( -13.14518615778179900, 35.14609375108393152, -5.444914386472297529 ) ) ;
#24639=CARTESIAN_POINT ( 'NONE',  ( -13.14518615778179544, 35.79101562608393294, 0.000000000000000000 ) ) ;
#24641=CARTESIAN_POINT ( 'NONE',  ( -13.57481594606304576, 34.74921875216787726, 0.000000000000000000 ) ) ;
#24653=DIRECTION ( 'NONE',  ( 1.374060148949977908E-06, 0.9999999999986906030, 8.549343071804204525E-07 ) ) ;
#24664=CARTESIAN_POINT ( 'NONE',  ( 13.14518615778179900, 37.13046875108393863, 5.444914386472293977 ) ) ;
#24675=CARTESIAN_POINT ( 'NONE',  ( -9.598844408820458085, 32.96328124999999432, -9.598844408820458085 ) ) ;
#24685=ORIENTED_EDGE ( 'NONE', *, *, #7420, .F. ) ;
#24687=DIRECTION ( 'NONE',  ( 0.000000000000000000, 0.000000000000000000, 1.000000000000000000 ) ) ;
#24695=CARTESIAN_POINT ( 'NONE',  ( 13.14518615778179544, 37.77539062608393294, -1.609821015232357215E-15 ) ) ;
#24712=CARTESIAN_POINT ( 'NONE',  ( 2.816687638038913930E-15, 21.95886589889650509, 23.00000000000001421 ) ) ;
#24737=ORIENTED_EDGE ( 'NONE', *, *, #14397, .F. ) ;
#24757=ADVANCED_FACE ( 'NONE', ( #24213 ), #19790, .T. ) ;
#24761=CARTESIAN_POINT ( 'NONE',  ( -13.14518615778179544, 32.81445312608393294, 0.000000000000000000 ) ) ;
#24764=CARTESIAN_POINT ( 'NONE',  ( -5.622872871577873077, 38.56914062716788294, -13.57481594606304753 ) ) ;
#24772=CARTESIAN_POINT ( 'NONE',  ( 2.493653234604083739E-15, 34.05468749999999289, 13.57481594606304576 ) ) ;
#24774=CARTESIAN_POINT ( 'NONE',  ( 9.295050272127047819, 33.11210937608393579, 9.295050272127046043 ) ) ;
#24776=CARTESIAN_POINT ( 'NONE',  ( 0.5696516875510663214, 35.99464330212366292, 13.14518615778179544 ) ) ;
#24777=CARTESIAN_POINT ( 'NONE',  ( 5.622872871577871301, 37.67617187716787441, -13.57481594606304753 ) ) ;
#24801=CARTESIAN_POINT ( 'NONE',  ( 13.14518615778179900, 34.84843750108393579, -5.444914386472297529 ) ) ;
#24817=DIRECTION ( 'NONE',  ( 0.000000000000000000, 1.000000000000000000, 0.000000000000000000 ) ) ;
#24834=CARTESIAN_POINT ( 'NONE',  ( 13.14518615778179900, 35.34453125108392868, 5.444914386472293977 ) ) ;
#24882=CARTESIAN_POINT ( 'NONE',  ( -13.57481594606304398, 35.59257812716789715, 5.622872871577880183 ) ) ;
#24905=CARTESIAN_POINT ( 'NONE',  ( 7.171391216998964424, 31.99955315621561525, -11.52591757658528948 ) ) ;
#24907=CARTESIAN_POINT ( 'NONE',  ( 2.493653234604083739E-15, 38.12265625216787157, 13.57481594606304576 ) ) ;
#24909=CARTESIAN_POINT ( 'NONE',  ( -8.312177448680279460E-16, 32.96328125216787441, -13.57481594606304576 ) ) ;
#24914=CARTESIAN_POINT ( 'NONE',  ( 13.57481594606304753, 34.30273437500000000, -5.622872871577873077 ) ) ;
#24915=CARTESIAN_POINT ( 'NONE',  ( -5.444914386472299306, 34.55078125108393294, 13.14518615778179722 ) ) ;
#24918=CARTESIAN_POINT ( 'NONE',  ( 13.57481594606304753, 37.57695312716787583, -5.622872871577873077 ) ) ;
#24922=DIRECTION ( 'NONE',  ( -0.000000000000000000, -1.000000000000000000, -0.000000000000000000 ) ) ;
#24941=CARTESIAN_POINT ( 'NONE',  ( -9.295050272127044266, 37.67617187608393436, 9.295050272127047819 ) ) ;
#24972=CARTESIAN_POINT ( 'NONE',  ( 13.14518615778179544, 36.18789062608393436, -1.609821015232357215E-15 ) ) ;
#25023=DIRECTION ( 'NONE',  ( 0.000000000000000000, 0.000000000000000000, 1.000000000000000000 ) ) ;
#25027=CARTESIAN_POINT ( 'NONE',  ( -13.14518615778179189, 39.21406250108392300, 5.444914386472304635 ) ) ;
#25043=CARTESIAN_POINT ( 'NONE',  ( -5.444914386472299306, 33.75703125108393721, 13.14518615778179722 ) ) ;
#25047=FILL_AREA_STYLE_COLOUR ( '', #6611 ) ;
#25055=CARTESIAN_POINT ( 'NONE',  ( -8.312177448680279460E-16, 34.45156249999999432, -13.57481594606304576 ) ) ;
#25057=CARTESIAN_POINT ( 'NONE',  ( -9.839381608887936892, 36.00000000000000711, -9.004033604613056241 ) ) ;
#25058=CARTESIAN_POINT ( 'NONE',  ( 2.493653234604083739E-15, 39.61093749999999147, 13.57481594606304576 ) ) ;
#25060=CARTESIAN_POINT ( 'NONE',  ( -9.295050272127046043, 34.10429687608393579, -9.295050272127046043 ) ) ;
#25062=CARTESIAN_POINT ( 'NONE',  ( -13.57481594606304753, 33.90585937716787868, -5.622872871577873077 ) ) ;
#25083=CARTESIAN_POINT ( 'NONE',  ( 5.444914386472297529, 34.15390625108393863, -13.14518615778179900 ) ) ;
#25113=CARTESIAN_POINT ( 'NONE',  ( -8.049105076161786076E-16, 33.21132812608393436, -13.14518615778179544 ) ) ;
#25125=CARTESIAN_POINT ( 'NONE',  ( 2.414731522848535132E-15, 36.78320312608393294, 13.14518615778179544 ) ) ;
#25147=CARTESIAN_POINT ( 'NONE',  ( 0.000000000000000000, 36.00000000000000000, 0.000000000000000000 ) ) ;
#25157=CARTESIAN_POINT ( 'NONE',  ( 5.444914386472297529, 40.50390625108394005, -13.14518615778179900 ) ) ;
#25176=EDGE_CURVE ( 'NONE', #12047, #25968, #20326, .T. ) ;
#25192=CARTESIAN_POINT ( 'NONE',  ( -4.459473413638155748, 36.00000000000000711, -12.68347323196786114 ) ) ;
#25193=CARTESIAN_POINT ( 'NONE',  ( 9.598844408820459861, 40.50390624999999289, 9.598844408820456309 ) ) ;
#25195=CARTESIAN_POINT ( 'NONE',  ( 9.295050272127046043, 33.11210937608393579, -9.295050272127046043 ) ) ;
#25197=CARTESIAN_POINT ( 'NONE',  ( 9.598844408820459861, 32.66562500216787157, 9.598844408820456309 ) ) ;
#25218=CARTESIAN_POINT ( 'NONE',  ( 13.14518615778179544, 34.00507812608393721, -1.609821015232357215E-15 ) ) ;
#25221=ADVANCED_FACE ( 'NONE', ( #7482 ), #16029, .T. ) ;
#25244=ORIENTED_EDGE ( 'NONE', *, *, #733, .T. ) ;
#25249=CARTESIAN_POINT ( 'NONE',  ( -8.049105076161786076E-16, 34.00507812608393721, -13.14518615778179544 ) ) ;
#25261=CARTESIAN_POINT ( 'NONE',  ( -9.295050272127046043, 35.69179687608393436, -9.295050272127046043 ) ) ;
#25293=DIRECTION ( 'NONE',  ( -0.000000000000000000, -1.000000000000000000, -0.000000000000000000 ) ) ;
#25298=CARTESIAN_POINT ( 'NONE',  ( -13.14518615778179900, 39.90859375108394147, -5.444914386472297529 ) ) ;
#25300=CIRCLE ( 'NONE', #13450, 22.40192378864669109 ) ;
#25304=VERTEX_POINT ( 'NONE', #10305 ) ;
#25316=CARTESIAN_POINT ( 'NONE',  ( 0.000000000000000000, 36.00000000000000000, -11.57481594606304576 ) ) ;
#25318=FILL_AREA_STYLE ('',( #25047 ) ) ;
#25325=ADVANCED_FACE ( 'NONE', ( #27725 ), #7871, .F. ) ;
#25331=CARTESIAN_POINT ( 'NONE',  ( 2.493653234604083739E-15, 40.40468749999999432, 13.57481594606304576 ) ) ;
#25332=CARTESIAN_POINT ( 'NONE',  ( -9.295050272127044266, 32.71523437608393436, 9.295050272127047819 ) ) ;
#25333=CARTESIAN_POINT ( 'NONE',  ( 2.493653234604083739E-15, 34.15390625216787157, 13.57481594606304576 ) ) ;
#25351=AXIS2_PLACEMENT_3D ( 'NONE', #16668, #27648, #23230 ) ;
#25362=CARTESIAN_POINT ( 'NONE',  ( 13.14518615778179900, 34.74921875108395142, 5.444914386472293977 ) ) ;
#25369=DIRECTION ( 'NONE',  ( 0.000000000000000000, 0.000000000000000000, -1.000000000000000000 ) ) ;
#25388=ORIENTED_EDGE ( 'NONE', *, *, #1321, .F. ) ;
#25395=CARTESIAN_POINT ( 'NONE',  ( 13.14518615778179544, 32.21914062608393436, -1.609821015232357215E-15 ) ) ;
#25404=DIRECTION ( 'NONE',  ( 0.000000000000000000, 1.000000000000000000, 0.000000000000000000 ) ) ;
#25410=CARTESIAN_POINT ( 'NONE',  ( -8.049105076161786076E-16, 34.00507812608393721, -13.14518615778179544 ) ) ;
#25418=CARTESIAN_POINT ( 'NONE',  ( 2.493653234604083739E-15, 31.77265625216787370, 13.57481594606304576 ) ) ;
#25471=CARTESIAN_POINT ( 'NONE',  ( -8.312177448680279460E-16, 32.07031249999999289, -13.57481594606304576 ) ) ;
#25472=VERTEX_POINT ( 'NONE', #24712 ) ;
#25474=CARTESIAN_POINT ( 'NONE',  ( -8.312177448680279460E-16, 40.80156249999999574, -13.57481594606304576 ) ) ;
#25475=CARTESIAN_POINT ( 'NONE',  ( 13.14518615778179722, 33.75703125108393010, 5.444914386472293977 ) ) ;
#25476=CARTESIAN_POINT ( 'NONE',  ( 13.57481594606304931, 33.50898437716787015, 5.622872871577869525 ) ) ;
#25494=VERTEX_POINT ( 'NONE', #9173 ) ;
#25497=CARTESIAN_POINT ( 'NONE',  ( 3.755639919285892248, 31.78804746655075419, -13.14518615778179544 ) ) ;
#25512=AXIS2_PLACEMENT_3D ( 'NONE', #18108, #13677, #5150 ) ;
#25525=VERTEX_POINT ( 'NONE', #27148 ) ;
#25530=CARTESIAN_POINT ( 'NONE',  ( -9.295050272127044266, 32.71523437608393436, 9.295050272127047819 ) ) ;
#25547=CARTESIAN_POINT ( 'NONE',  ( -13.14518615778179189, 31.87187500108393223, 5.444914386472304635 ) ) ;
#25567=CARTESIAN_POINT ( 'NONE',  ( -8.312177448680279460E-16, 32.16953125216787157, -13.57481594606304576 ) ) ;
#25574=CARTESIAN_POINT ( 'NONE',  ( 5.622872871577780707, 33.70742187716788152, -13.57481594606313990 ) ) ;
#25576=CARTESIAN_POINT ( 'NONE',  ( 2.493653234604083739E-15, 34.15390625216787157, 13.57481594606304576 ) ) ;
#25582=ORIENTED_EDGE ( 'NONE', *, *, #26376, .F. ) ;
#25603=CARTESIAN_POINT ( 'NONE',  ( -5.444914386472297529, 31.87187500108393223, -13.14518615778179900 ) ) ;
#25604=CARTESIAN_POINT ( 'NONE',  ( -5.444914386472299306, 31.97109375108393792, 13.14518615778179722 ) ) ;
#25606=CARTESIAN_POINT ( 'NONE',  ( 9.598844408820456309, 33.65781250216787157, -9.598844408820458085 ) ) ;
#25646=CARTESIAN_POINT ( 'NONE',  ( 1.417506129906585201E-15, 36.00000000000000000, 11.57481594606304576 ) ) ;
#25651=AXIS2_PLACEMENT_3D ( 'NONE', #27475, #18499, #16628 ) ;
#25657=ORIENTED_EDGE ( 'NONE', *, *, #984, .F. ) ;
#25661=CARTESIAN_POINT ( 'NONE',  ( 5.444914386472302859, 34.65000000108393863, 13.14518615778179189 ) ) ;
#25663=CARTESIAN_POINT ( 'NONE',  ( 5.444914386472297529, 32.36796875108393579, -13.14518615778179900 ) ) ;
#25675=AXIS2_PLACEMENT_3D ( 'NONE', #14801, #12520, #12802 ) ;
#25678=DIRECTION ( 'NONE',  ( 0.000000000000000000, 1.000000000000000000, 0.000000000000000000 ) ) ;
#25701=( BOUNDED_CURVE ( )  B_SPLINE_CURVE ( 1, ( #27064, #15492 ),
 .UNSPECIFIED., .F., .F. ) 
 B_SPLINE_CURVE_WITH_KNOTS ( ( 2, 2 ),
 ( 0.000000000000000000, 1.000000000000000000 ),
 .UNSPECIFIED. ) 
 CURVE ( )  GEOMETRIC_REPRESENTATION_ITEM ( )  RATIONAL_B_SPLINE_CURVE ( ( 0.9684275698016389100, 0.9684275698016389100 ) ) 
 REPRESENTATION_ITEM ( '' )  );
#25732=AXIS2_PLACEMENT_3D ( 'NONE', #4884, #21847, #26402 ) ;
#25738=SHAPE_REPRESENTATION_RELATIONSHIP ( 'NONE' , 'NONE' ,  #9145, #11047 ) ;
#25741=CARTESIAN_POINT ( 'NONE',  ( -13.57481594606304753, 32.21914062500000142, -5.622872871577873077 ) ) ;
#25744=DIRECTION ( 'NONE',  ( -0.000000000000000000, -1.000000000000000000, -0.000000000000000000 ) ) ;
#25746=CARTESIAN_POINT ( 'NONE',  ( 5.444914386472302859, 33.65781250108393152, 13.14518615778179189 ) ) ;
#25747=CARTESIAN_POINT ( 'NONE',  ( -5.444914386472297529, 40.40468750108393436, -13.14518615778179900 ) ) ;
#25772=CARTESIAN_POINT ( 'NONE',  ( 9.598844408820456309, 35.93984374999999432, -9.598844408820458085 ) ) ;
#25796=EDGE_LOOP ( 'NONE', ( #2825, #14984, #19190, #16685 ) ) ;
#25801=CARTESIAN_POINT ( 'NONE',  ( 9.295050272127047819, 34.69960937608393436, 9.295050272127046043 ) ) ;
#25802=CARTESIAN_POINT ( 'NONE',  ( 5.444914386472302859, 40.20625000108394431, 13.14518615778179189 ) ) ;
#25822=CARTESIAN_POINT ( 'NONE',  ( -13.14518615778179189, 33.45937500108392726, 5.444914386472304635 ) ) ;
#25849=ORIENTED_EDGE ( 'NONE', *, *, #1836, .T. ) ;
#25893=CARTESIAN_POINT ( 'NONE',  ( -13.14518615778179900, 39.71015625108393010, -5.444914386472297529 ) ) ;
#25918=CARTESIAN_POINT ( 'NONE',  ( 2.493653234604083739E-15, 35.64218749999999147, 13.57481594606304576 ) ) ;
#25922=CARTESIAN_POINT ( 'NONE',  ( 2.414731522848535132E-15, 37.77539062608393294, 13.14518615778179544 ) ) ;
#25946=CARTESIAN_POINT ( 'NONE',  ( 3.755639919285892248, 31.58960996655074993, -13.14518615778179544 ) ) ;
#25965=CARTESIAN_POINT ( 'NONE',  ( -5.444914386472297529, 34.05468750108393294, -13.14518615778179900 ) ) ;
#25968=VERTEX_POINT ( 'NONE', #26615 ) ;
#25982=CARTESIAN_POINT ( 'NONE',  ( -5.444914386472297529, 38.81718750108393579, -13.14518615778179900 ) ) ;
#25985=DIRECTION ( 'NONE',  ( 0.000000000000000000, 0.000000000000000000, 1.000000000000000000 ) ) ;
#26000=CYLINDRICAL_SURFACE ( 'NONE', #1820, 13.57481594606304576 ) ;
#26014=CARTESIAN_POINT ( 'NONE',  ( -9.295050272127044266, 33.70742187608393436, 9.295050272127047819 ) ) ;
#26026=CARTESIAN_POINT ( 'NONE',  ( 5.444914386472297529, 40.30546875108393579, -13.14518615778179900 ) ) ;
#26035=CARTESIAN_POINT ( 'NONE',  ( 6.944426393311537993, 31.75150625057403175, -11.16113171639042356 ) ) ;
#26045=CARTESIAN_POINT ( 'NONE',  ( 13.04200858114962713, 35.99999999999998579, -3.640726557254823081 ) ) ;
#26057=CARTESIAN_POINT ( 'NONE',  ( -9.598844408820458085, 37.72578124999999005, -9.598844408820458085 ) ) ;
#26059=CARTESIAN_POINT ( 'NONE',  ( -5.444914386472299306, 38.51953125108393294, 13.14518615778179722 ) ) ;
#26085=CARTESIAN_POINT ( 'NONE',  ( 13.14518615778179722, 34.05468750108394005, -5.444914386472297529 ) ) ;
#26086=CARTESIAN_POINT ( 'NONE',  ( 13.14518615778179900, 39.61093750108393863, -5.444914386472297529 ) ) ;
#26087=UNCERTAINTY_MEASURE_WITH_UNIT (LENGTH_MEASURE( 1.000000000000000082E-05 ), #4325, 'distance_accuracy_value', 'NONE');
#26120=CARTESIAN_POINT ( 'NONE',  ( -13.14518615778179900, 38.91640625108393436, -5.444914386472297529 ) ) ;
#26162=LINE ( 'NONE', #17325, #3174 ) ;
#26168=CARTESIAN_POINT ( 'NONE',  ( 13.14518615778179900, 38.51953125108393294, 5.444914386472293977 ) ) ;
#26197=CARTESIAN_POINT ( 'NONE',  ( -13.57481594606304576, 32.36796875216787583, 0.000000000000000000 ) ) ;
#26198=CARTESIAN_POINT ( 'NONE',  ( 5.622872871577871301, 36.78320312499999289, -13.57481594606304753 ) ) ;
#26201=CARTESIAN_POINT ( 'NONE',  ( 9.295050272127046043, 38.07304687608393579, -9.295050272127046043 ) ) ;
#26220=AXIS2_PLACEMENT_3D ( 'NONE', #4100, #24182, #6505 ) ;
#26230=CARTESIAN_POINT ( 'NONE',  ( -5.444914386472297529, 35.84062500108394289, -13.14518615778179722 ) ) ;
#26231=CARTESIAN_POINT ( 'NONE',  ( -8.049105076161786076E-16, 38.17226562608394147, -13.14518615778179544 ) ) ;
#26262=DIRECTION ( 'NONE',  ( 0.000000000000000000, 1.000000000000000000, 0.000000000000000000 ) ) ;
#26266=CARTESIAN_POINT ( 'NONE',  ( 2.414731522848535132E-15, 39.16445312608392726, 13.14518615778179544 ) ) ;
#26271=CLOSED_SHELL ( 'NONE', ( #14818, #21019, #17599, #25325, #27632, #7925, #3241, #16277, #18123, #13474, #7933, #24757, #5528, #10565, #26406, #5704, #6907, #15699, #12774, #27763, #6504, #24157, #11890, #23258, #1138, #4857, #25221, #3527, #18200, #22194, #14012, #13999, #19772, #20306, #16657, #10371, #1364, #26865, #19086 ) ) ;
#26293=CIRCLE ( 'NONE', #5369, 24.13397459621556962 ) ;
#26307=CARTESIAN_POINT ( 'NONE',  ( 2.816687638038913930E-15, 23.00000000000000000, 23.00000000000001421 ) ) ;
#26316=CARTESIAN_POINT ( 'NONE',  ( 13.14518615778179900, 39.41250000108393436, -5.444914386472297529 ) ) ;
#26323=DIRECTION ( 'NONE',  ( 0.000000000000000000, 0.000000000000000000, -1.000000000000000000 ) ) ;
#26327=VERTEX_POINT ( 'NONE', #11445 ) ;
#26348=CARTESIAN_POINT ( 'NONE',  ( -8.312177448680279460E-16, 38.42031249999999432, -13.57481594606304576 ) ) ;
#26349=CARTESIAN_POINT ( 'NONE',  ( -1.271138771240642784, 36.00000000000000000, -13.43002483374384681 ) ) ;
#26350=CARTESIAN_POINT ( 'NONE',  ( -5.444914386472297529, 39.01562500108394005, -13.14518615778179900 ) ) ;
#26376=EDGE_CURVE ( 'NONE', #11554, #19382, #6969, .T. ) ;
#26379=CARTESIAN_POINT ( 'NONE',  ( 5.444914386472297529, 40.50390625108394005, -13.14518615778179900 ) ) ;
#26402=DIRECTION ( 'NONE',  ( 0.000000000000000000, 0.000000000000000000, -1.000000000000000000 ) ) ;
#26405=ORIENTED_EDGE ( 'NONE', *, *, #4266, .F. ) ;
#26406=ADVANCED_FACE ( 'NONE', ( #19284 ), #41, .T. ) ;
#26412=CARTESIAN_POINT ( 'NONE',  ( -9.295050272127044266, 39.06523437608392868, 9.295050272127047819 ) ) ;
#26422=( BOUNDED_CURVE ( )  B_SPLINE_CURVE ( 2, ( #18257, #17683, #22536, #21971, #24527, #5012, #11109, #24242, #19823 ),
 .UNSPECIFIED., .F., .F. ) 
 B_SPLINE_CURVE_WITH_KNOTS ( ( 3, 2, 2, 2, 3 ),
 ( 0.6458333333333333703, 0.6562500000000000000, 0.6666666666666665186, 0.6770833333333332593, 0.6874999999999997780 ),
 .UNSPECIFIED. ) 
 CURVE ( )  GEOMETRIC_REPRESENTATION_ITEM ( )  RATIONAL_B_SPLINE_CURVE ( ( 1.000000000000000000, 0.9238795325112867385, 1.000000000000000000, 0.9238795325112867385, 1.000000000000000000, 0.9238795325112867385, 1.000000000000000000, 0.9238795325112884038, 0.9999999999999983347 ) ) 
 REPRESENTATION_ITEM ( '' )  );
#26462=CARTESIAN_POINT ( 'NONE',  ( 9.295050272127046043, 34.69960937608393436, -9.295050272127046043 ) ) ;
#26485=CARTESIAN_POINT ( 'NONE',  ( 13.57481594606304576, 38.32109375216786873, -1.662435489736055892E-15 ) ) ;
#26492=CARTESIAN_POINT ( 'NONE',  ( -13.57481594606304576, 38.66835937499999432, 5.622872871577880183 ) ) ;
#26494=CARTESIAN_POINT ( 'NONE',  ( 5.444914386472297529, 38.91640625108393436, -13.14518615778179900 ) ) ;
#26504=DIRECTION ( 'NONE',  ( 0.000000000000000000, 0.8660254037844380415, 0.5000000000000009992 ) ) ;
#26520=CARTESIAN_POINT ( 'NONE',  ( 13.14518615778179544, 35.59257812608393579, -1.609821015232357215E-15 ) ) ;
#26544=DIRECTION ( 'NONE',  ( 0.000000000000000000, -0.5735764363510443831, 0.8191520442889929088 ) ) ;
#26550=EDGE_LOOP ( 'NONE', ( #27174, #20415, #9886, #14458 ) ) ;
#26552=CARTESIAN_POINT ( 'NONE',  ( 5.444914386472302859, 40.00781250108393294, 13.14518615778179189 ) ) ;
#26554=AXIS2_PLACEMENT_3D ( 'NONE', #23702, #24122, #23839 ) ;
#26575=CARTESIAN_POINT ( 'NONE',  ( 13.57481594606304576, 34.25312499999999716, -1.662435489736055892E-15 ) ) ;
#26601=ORIENTED_EDGE ( 'NONE', *, *, #25176, .F. ) ;
#26606=CARTESIAN_POINT ( 'NONE',  ( 5.444914386472297529, 37.13046875108393152, -13.14518615778179900 ) ) ;
#26608=DIRECTION ( 'NONE',  ( -0.000000000000000000, -1.000000000000000000, -0.000000000000000000 ) ) ;
#26615=CARTESIAN_POINT ( 'NONE',  ( -8.312177448680279460E-16, 35.24531249999999716, -13.57481594606304576 ) ) ;
#26619=ORIENTED_EDGE ( 'NONE', *, *, #11748, .F. ) ;
#26630=AXIS2_PLACEMENT_3D ( 'NONE', #19316, #6481, #14879 ) ;
#26631=CARTESIAN_POINT ( 'NONE',  ( 13.57481594606304753, 39.16445312716788152, -5.622872871577873077 ) ) ;
#26635=FACE_OUTER_BOUND ( 'NONE', #15084, .T. ) ;
#26638=CARTESIAN_POINT ( 'NONE',  ( -13.57481594606304753, 38.56914062500000284, -5.622872871577873077 ) ) ;
#26640=CARTESIAN_POINT ( 'NONE',  ( -9.295050272127044266, 32.91367187608393152, 9.295050272127047819 ) ) ;
#26643=CARTESIAN_POINT ( 'NONE',  ( 5.622872871577871301, 36.88242187716787157, -13.57481594606304753 ) ) ;
#26666=VERTEX_POINT ( 'NONE', #21435 ) ;
#26667=CARTESIAN_POINT ( 'NONE',  ( 13.14518615778179544, 36.38632812608393863, -1.609821015232357215E-15 ) ) ;
#26697=CARTESIAN_POINT ( 'NONE',  ( 5.444914386472297529, 37.13046875108393152, -13.14518615778179900 ) ) ;
#26748=CARTESIAN_POINT ( 'NONE',  ( 2.414731522848535132E-15, 34.40195312608393152, 13.14518615778179544 ) ) ;
#26752=CARTESIAN_POINT ( 'NONE',  ( -13.14518615778179544, 40.75195312608393294, 0.000000000000000000 ) ) ;
#26754=AXIS2_PLACEMENT_3D ( 'NONE', #2683, #13192, #2818 ) ;
#26773=CARTESIAN_POINT ( 'NONE',  ( -5.622872871577873077, 39.66054687716786731, 13.57481594606304753 ) ) ;
#26776=CARTESIAN_POINT ( 'NONE',  ( -9.598844408820458085, 33.06250000216787299, -9.598844408820458085 ) ) ;
#26782=CARTESIAN_POINT ( 'NONE',  ( -13.57481594606304576, 33.85624999999999574, 0.000000000000000000 ) ) ;
#26784=CARTESIAN_POINT ( 'NONE',  ( -8.049105076161786076E-16, 35.79101562608394005, -13.14518615778179544 ) ) ;
#26786=CARTESIAN_POINT ( 'NONE',  ( -5.444914386472299306, 35.14609375108393152, 13.14518615778179722 ) ) ;
#26787=CARTESIAN_POINT ( 'NONE',  ( -13.57481594606304576, 34.79882812716787299, 5.622872871577880183 ) ) ;
#26811=CARTESIAN_POINT ( 'NONE',  ( 9.295050272127046043, 35.69179687608394147, -9.295050272127046043 ) ) ;
#26816=CARTESIAN_POINT ( 'NONE',  ( 0.000000000000000000, 0.000000000000000000, 0.000000000000000000 ) ) ;
#26822=AXIS2_PLACEMENT_3D ( 'NONE', #21820, #11381, #19808 ) ;
#26834=EDGE_LOOP ( 'NONE', ( #17821, #27127, #9710, #1870 ) ) ;
#26841=ORIENTED_EDGE ( 'NONE', *, *, #21090, .T. ) ;
#26843=CARTESIAN_POINT ( 'NONE',  ( 13.14518615778179900, 36.93203125108394147, 5.444914386472293977 ) ) ;
#26844=AXIS2_PLACEMENT_3D ( 'NONE', #8635, #24028, #23608 ) ;
#26858=EDGE_LOOP ( 'NONE', ( #3282, #13467, #16952, #8102 ) ) ;
#26865=ADVANCED_FACE ( 'NONE', ( #9157 ), #21885, .T. ) ;
#26892=CARTESIAN_POINT ( 'NONE',  ( 5.444914386472302859, 36.83281250108392868, 13.14518615778179189 ) ) ;
#26899=PLANE ( 'NONE',  #18610 ) ;
#26913=CARTESIAN_POINT ( 'NONE',  ( 9.295050272127047819, 33.11210937608393579, 9.295050272127046043 ) ) ;
#26917=CARTESIAN_POINT ( 'NONE',  ( -13.57481594606304576, 39.56132812716787583, 5.622872871577880183 ) ) ;
#26926=CARTESIAN_POINT ( 'NONE',  ( -9.598844408820454532, 33.95546874999999432, 9.598844408820459861 ) ) ;
#26928=CARTESIAN_POINT ( 'NONE',  ( -9.295050272127046043, 33.50898437608393010, -9.295050272127046043 ) ) ;
#26931=CARTESIAN_POINT ( 'NONE',  ( -13.57481594606304576, 37.18007812716787441, 5.622872871577880183 ) ) ;
#26957=CARTESIAN_POINT ( 'NONE',  ( 9.295050272127047819, 37.08085937608393579, 9.295050272127046043 ) ) ;
#26987=CARTESIAN_POINT ( 'NONE',  ( 13.14518615778179900, 37.03125000108393294, -5.444914386472297529 ) ) ;
#27010=VERTEX_POINT ( 'NONE', #4356 ) ;
#27053=CARTESIAN_POINT ( 'NONE',  ( -5.444914386472297529, 31.87187500108393223, -13.14518615778179722 ) ) ;
#27058=CARTESIAN_POINT ( 'NONE',  ( -5.622872871577873077, 39.36289062716787157, -13.57481594606304753 ) ) ;
#27062=DIRECTION ( 'NONE',  ( 0.000000000000000000, 0.000000000000000000, -1.000000000000000000 ) ) ;
#27064=CARTESIAN_POINT ( 'NONE',  ( 7.171391216998964424, 31.99955315621561525, -11.52591757658528948 ) ) ;
#27066=CARTESIAN_POINT ( 'NONE',  ( -5.622872871577873077, 34.50117187499999005, -13.57481594606304753 ) ) ;
#27067=CARTESIAN_POINT ( 'NONE',  ( -2.892062521303301548, 36.00000000000000711, -13.15766692561478024 ) ) ;
#27068=CARTESIAN_POINT ( 'NONE',  ( 9.295050272127047819, 34.69960937608393436, 9.295050272127046043 ) ) ;
#27070=CARTESIAN_POINT ( 'NONE',  ( 5.444914386472302859, 34.45156250108392726, 13.14518615778179189 ) ) ;
#27071=CARTESIAN_POINT ( 'NONE',  ( 13.57481594606304753, 35.98945312716787015, -5.622872871577873077 ) ) ;
#27072=CARTESIAN_POINT ( 'NONE',  ( 0.000000000000000000, 36.00000000000000000, -13.57481594606304576 ) ) ;
#27095=CARTESIAN_POINT ( 'NONE',  ( -8.049105076161786076E-16, 36.58476562608393579, -13.14518615778179544 ) ) ;
#27119=FACE_OUTER_BOUND ( 'NONE', #20376, .T. ) ;
#27127=ORIENTED_EDGE ( 'NONE', *, *, #18490, .T. ) ;
#27130=CARTESIAN_POINT ( 'NONE',  ( -13.14518615778179189, 35.84062500108394289, 5.444914386472304635 ) ) ;
#27138=LINE ( 'NONE', #1199, #22831 ) ;
#27148=CARTESIAN_POINT ( 'NONE',  ( 4.157286354961724939, 36.00000000000000000, -12.92256159328856135 ) ) ;
#27168=EDGE_CURVE ( 'NONE', #12136, #13023, #27729, .T. ) ;
#27174=ORIENTED_EDGE ( 'NONE', *, *, #18883, .T. ) ;
#27186=CARTESIAN_POINT ( 'NONE',  ( 7.171390501253594785, 31.30502191632583830, -11.52591802191987114 ) ) ;
#27207=CARTESIAN_POINT ( 'NONE',  ( 0.000000000000000000, 36.00000000000000000, 0.000000000000000000 ) ) ;
#27210=CARTESIAN_POINT ( 'NONE',  ( 5.622872871577878406, 34.89804687499999147, 13.57481594606304576 ) ) ;
#27211=CARTESIAN_POINT ( 'NONE',  ( 5.622872871577871301, 39.95820312499999716, -13.57481594606304753 ) ) ;
#27214=CARTESIAN_POINT ( 'NONE',  ( 13.57481594606304931, 35.09648437716787583, 5.622872871577869525 ) ) ;
#27237=CARTESIAN_POINT ( 'NONE',  ( 13.14518615778179544, 32.41757812608393863, -1.609821015232357215E-15 ) ) ;
#27239=CARTESIAN_POINT ( 'NONE',  ( 5.622872871577832221, 35.79101562716787299, 13.57481594606309194 ) ) ;
#27258=DIRECTION ( 'NONE',  ( 0.000000000000000000, 0.000000000000000000, 1.000000000000000000 ) ) ;
#27259=PRODUCT_DEFINITION_FORMATION_WITH_SPECIFIED_SOURCE ( 'ANY', '', #16047, .NOT_KNOWN. ) ;
#27268=CARTESIAN_POINT ( 'NONE',  ( 5.444914386472297529, 34.74921875108394431, -13.14518615778179900 ) ) ;
#27308=DIRECTION ( 'NONE',  ( 0.000000000000000000, 0.000000000000000000, 1.000000000000000000 ) ) ;
#27315=AXIS2_PLACEMENT_3D ( 'NONE', #11834, #11407, #5305 ) ;
#27318=LINE ( 'NONE', #5647, #2714 ) ;
#27319=CARTESIAN_POINT ( 'NONE',  ( 5.444914386472302859, 40.20625000108394431, 13.14518615778179189 ) ) ;
#27347=CARTESIAN_POINT ( 'NONE',  ( 5.622872871577878406, 32.51679687499999716, 13.57481594606304576 ) ) ;
#27350=CARTESIAN_POINT ( 'NONE',  ( 9.598844408820456309, 39.90859374999999432, -9.598844408820458085 ) ) ;
#27352=CARTESIAN_POINT ( 'NONE',  ( 5.444914386472297529, 35.54296875108393294, -13.14518615778179722 ) ) ;
#27353=CARTESIAN_POINT ( 'NONE',  ( -5.622872871577873077, 33.31054687716787299, 13.57481594606304753 ) ) ;
#27357=( BOUNDED_CURVE ( )  B_SPLINE_CURVE ( 2, ( #12007, #1215, #9880, #18588, #9411, #16397, #24675, #1029, #9700 ),
 .UNSPECIFIED., .F., .F. ) 
 B_SPLINE_CURVE_WITH_KNOTS ( ( 3, 2, 2, 2, 3 ),
 ( 0.8124999999999998890, 0.8229166666666665186, 0.8333333333333331483, 0.8437499999999997780, 0.8541666666666662966 ),
 .UNSPECIFIED. ) 
 CURVE ( )  GEOMETRIC_REPRESENTATION_ITEM ( )  RATIONAL_B_SPLINE_CURVE ( ( 1.000000000000000888, 0.9238795325112859613, 1.000000000000000000, 0.9238795325112867385, 1.000000000000000000, 0.9238795325112867385, 1.000000000000000000, 0.9238795325112891810, 0.9999999999999975575 ) ) 
 REPRESENTATION_ITEM ( '' )  );
#27363=ORIENTED_EDGE ( 'NONE', *, *, #8596, .T. ) ;
#27373=CARTESIAN_POINT ( 'NONE',  ( 5.444914386472297529, 33.36015625108393579, -13.14518615778179900 ) ) ;
#27403=CARTESIAN_POINT ( 'NONE',  ( -9.295050272127044266, 31.92148437608393508, 9.295050272127047819 ) ) ;
#27413=CARTESIAN_POINT ( 'NONE',  ( -13.14518615778179544, 34.99726562608393721, 0.000000000000000000 ) ) ;
#27449=CARTESIAN_POINT ( 'NONE',  ( -8.049105076161786076E-16, 40.55351562608393579, -13.14518615778179544 ) ) ;
#27475=CARTESIAN_POINT ( 'NONE',  ( 0.000000000000000000, 36.00000000000000000, 0.000000000000000000 ) ) ;
#27480=EDGE_CURVE ( 'NONE', #18468, #19839, #28167, .T. ) ;
#27481=CARTESIAN_POINT ( 'NONE',  ( 2.493653234604083739E-15, 32.56640625216787299, 13.57481594606304576 ) ) ;
#27483=CARTESIAN_POINT ( 'NONE',  ( 7.171391216998965312, 31.99955315621561525, -11.52591757658528948 ) ) ;
#27486=CARTESIAN_POINT ( 'NONE',  ( -13.14518615778179189, 32.07031250108393294, 5.444914386472304635 ) ) ;
#27488=CARTESIAN_POINT ( 'NONE',  ( -13.57481594606304576, 31.57421875216786944, 0.000000000000000000 ) ) ;
#27508=EDGE_LOOP ( 'NONE', ( #25388, #16796, #5905, #22381 ) ) ;
#27509=CARTESIAN_POINT ( 'NONE',  ( -13.14518615778179189, 34.45156250108394147, 5.444914386472304635 ) ) ;
#27528=CARTESIAN_POINT ( 'NONE',  ( -13.05838185645087357, 36.00000000000000711, 1.569311539113942500 ) ) ;
#27540=CARTESIAN_POINT ( 'NONE',  ( 5.444914386472297529, 33.16171875108393152, -13.14518615778179900 ) ) ;
#27555=CARTESIAN_POINT ( 'NONE',  ( 2.414731522848535132E-15, 33.60820312608392868, 13.14518615778179544 ) ) ;
#27557=ORIENTED_EDGE ( 'NONE', *, *, #12380, .T. ) ;
#27559=CYLINDRICAL_SURFACE ( 'NONE', #17059, 13.57481594606304576 ) ;
#27587=CARTESIAN_POINT ( 'NONE',  ( 0.000000000000000000, 21.36169591142201440, 0.000000000000000000 ) ) ;
#27603=VECTOR ( 'NONE', #24922, 1000.000000000000000 ) ;
#27611=FACE_BOUND ( 'NONE', #5883, .T. ) ;
#27621=CARTESIAN_POINT ( 'NONE',  ( 6.944423624769117787, 31.75150628229955529, -11.16113343896966370 ) ) ;
#27623=CARTESIAN_POINT ( 'NONE',  ( -5.622872871577873077, 31.42539062716787157, -13.57481594606304753 ) ) ;
#27632=ADVANCED_FACE ( 'NONE', ( #13636 ), #5251, .F. ) ;
#27642=EDGE_CURVE ( 'NONE', #15131, #25968, #19707, .T. ) ;
#27644=EDGE_LOOP ( 'NONE', ( #12851, #6596, #15799, #7962 ) ) ;
#27645=CARTESIAN_POINT ( 'NONE',  ( -5.444914386472297529, 32.66562500108393863, -13.14518615778179900 ) ) ;
#27648=DIRECTION ( 'NONE',  ( 0.000000000000000000, 1.000000000000000000, 0.000000000000000000 ) ) ;
#27662=CARTESIAN_POINT ( 'NONE',  ( -2.297960586007286476, 36.00000000000000000, 12.97104423350697466 ) ) ;
#27677=CARTESIAN_POINT ( 'NONE',  ( -9.295050272127044266, 34.30273437608393294, 9.295050272127047819 ) ) ;
#27694=CARTESIAN_POINT ( 'NONE',  ( 5.444914386472297529, 33.16171875108393152, -13.14518615778179900 ) ) ;
#27725=FACE_OUTER_BOUND ( 'NONE', #2467, .T. ) ;
#27729=CIRCLE ( 'NONE', #13121, 13.57481594606304576 ) ;
#27756=CARTESIAN_POINT ( 'NONE',  ( -13.14518615778179900, 31.97109375108393436, -5.444914386472297529 ) ) ;
#27757=CARTESIAN_POINT ( 'NONE',  ( -8.049105076161786076E-16, 32.41757812608393863, -13.14518615778179544 ) ) ;
#27759=CARTESIAN_POINT ( 'NONE',  ( 13.57481594606304576, 33.55859375216787299, -1.662435489736055892E-15 ) ) ;
#27763=ADVANCED_FACE ( 'NONE', ( #20210 ), #4831, .T. ) ;
#27776=DIRECTION ( 'NONE',  ( 0.000000000000000000, -0.5735764363510443831, 0.8191520442889929088 ) ) ;
#27798=EDGE_CURVE ( 'NONE', #21990, #22337, #25701, .T. ) ;
#27818=CARTESIAN_POINT ( 'NONE',  ( 2.414731522848535132E-15, 34.60039062608393579, 13.14518615778179544 ) ) ;
#27819=CARTESIAN_POINT ( 'NONE',  ( 9.295050272127046043, 33.11210937608393579, -9.295050272127046043 ) ) ;
#27835=CARTESIAN_POINT ( 'NONE',  ( 13.14518615778179900, 32.26875000108393721, -5.444914386472297529 ) ) ;
#27857=VERTEX_POINT ( 'NONE', #27481 ) ;
#27858=ORIENTED_EDGE ( 'NONE', *, *, #3745, .F. ) ;
#27864=CARTESIAN_POINT ( 'NONE',  ( -3.061616997868384226E-15, 23.00000000000000000, -25.00000000000001066 ) ) ;
#27877=ORIENTED_EDGE ( 'NONE', *, *, #5353, .T. ) ;
#27881=CARTESIAN_POINT ( 'NONE',  ( 0.000000000000000000, 11.00000000000000355, 17.49444650053485972 ) ) ;
#27888=( NAMED_UNIT ( * ) SI_UNIT ( $, .STERADIAN. ) SOLID_ANGLE_UNIT ( ) );
#27895=CARTESIAN_POINT ( 'NONE',  ( -13.14518615778179544, 32.61601562608393579, 0.000000000000000000 ) ) ;
#27897=CARTESIAN_POINT ( 'NONE',  ( 2.493653234604083739E-15, 31.77265625216787370, 13.57481594606304576 ) ) ;
#27923=CARTESIAN_POINT ( 'NONE',  ( 13.57481594606304931, 35.79101562499999289, 5.622872871577868636 ) ) ;
#27951=ORIENTED_EDGE ( 'NONE', *, *, #6682, .F. ) ;
#27953=CARTESIAN_POINT ( 'NONE',  ( 9.295050272127046043, 39.66054687608393436, -9.295050272127046043 ) ) ;
#27970=CARTESIAN_POINT ( 'NONE',  ( 0.000000000000000000, 10.00000000000000000, 0.000000000000000000 ) ) ;
#27971=CARTESIAN_POINT ( 'NONE',  ( -5.444914386472299306, 31.97109375108393436, 13.14518615778179722 ) ) ;
#27975=DIRECTION ( 'NONE',  ( -0.000000000000000000, -1.000000000000000000, -0.000000000000000000 ) ) ;
#28034=CARTESIAN_POINT ( 'NONE',  ( 2.414731522848535132E-15, 38.37070312608393152, 13.14518615778179544 ) ) ;
#28043=CARTESIAN_POINT ( 'NONE',  ( 6.944423797152706079, 31.55306878032414986, -11.16113333171310451 ) ) ;
#28052=CARTESIAN_POINT ( 'NONE',  ( 12.32011696698886816, 36.00000000000002842, -5.704949255836476496 ) ) ;
#28065=CARTESIAN_POINT ( 'NONE',  ( -13.14518615778179544, 36.78320312608393294, 0.000000000000000000 ) ) ;
#28075=AXIS2_PLACEMENT_3D ( 'NONE', #9225, #22346, #9085 ) ;
#28076=CARTESIAN_POINT ( 'NONE',  ( -4.374022130817611931, 35.99999999999999289, 12.40367315690591887 ) ) ;
#28092=CARTESIAN_POINT ( 'NONE',  ( -13.14518615778179544, 39.95820312608393010, 0.000000000000000000 ) ) ;
#28108=AXIS2_PLACEMENT_3D ( 'NONE', #4428, #13370, #11238 ) ;
#28110=CARTESIAN_POINT ( 'NONE',  ( 6.944423797152705191, 31.55306878032414986, -11.16113333171310451 ) ) ;
#28125=CARTESIAN_POINT ( 'NONE',  ( 13.14518615778179544, 39.36289062608393152, -1.609821015232357215E-15 ) ) ;
#28143=DIRECTION ( 'NONE',  ( -0.000000000000000000, -1.000000000000000000, -0.000000000000000000 ) ) ;
#28153=EDGE_CURVE ( 'NONE', #11809, #13376, #26162, .T. ) ;
#28159=CARTESIAN_POINT ( 'NONE',  ( -8.049105076161786076E-16, 33.40976562608393863, -13.14518615778179544 ) ) ;
#28162=ORIENTED_EDGE ( 'NONE', *, *, #22456, .T. ) ;
#28167=CIRCLE ( 'NONE', #11773, 16.91709623134523000 ) ;
#28172=CARTESIAN_POINT ( 'NONE',  ( 2.414731522848535132E-15, 39.16445312608392726, 13.14518615778179544 ) ) ;
#28202=CARTESIAN_POINT ( 'NONE',  ( 13.57481594606304931, 38.17226562499999432, 5.622872871577869525 ) ) ;
ENDSEC;
END-ISO-10303-21;
